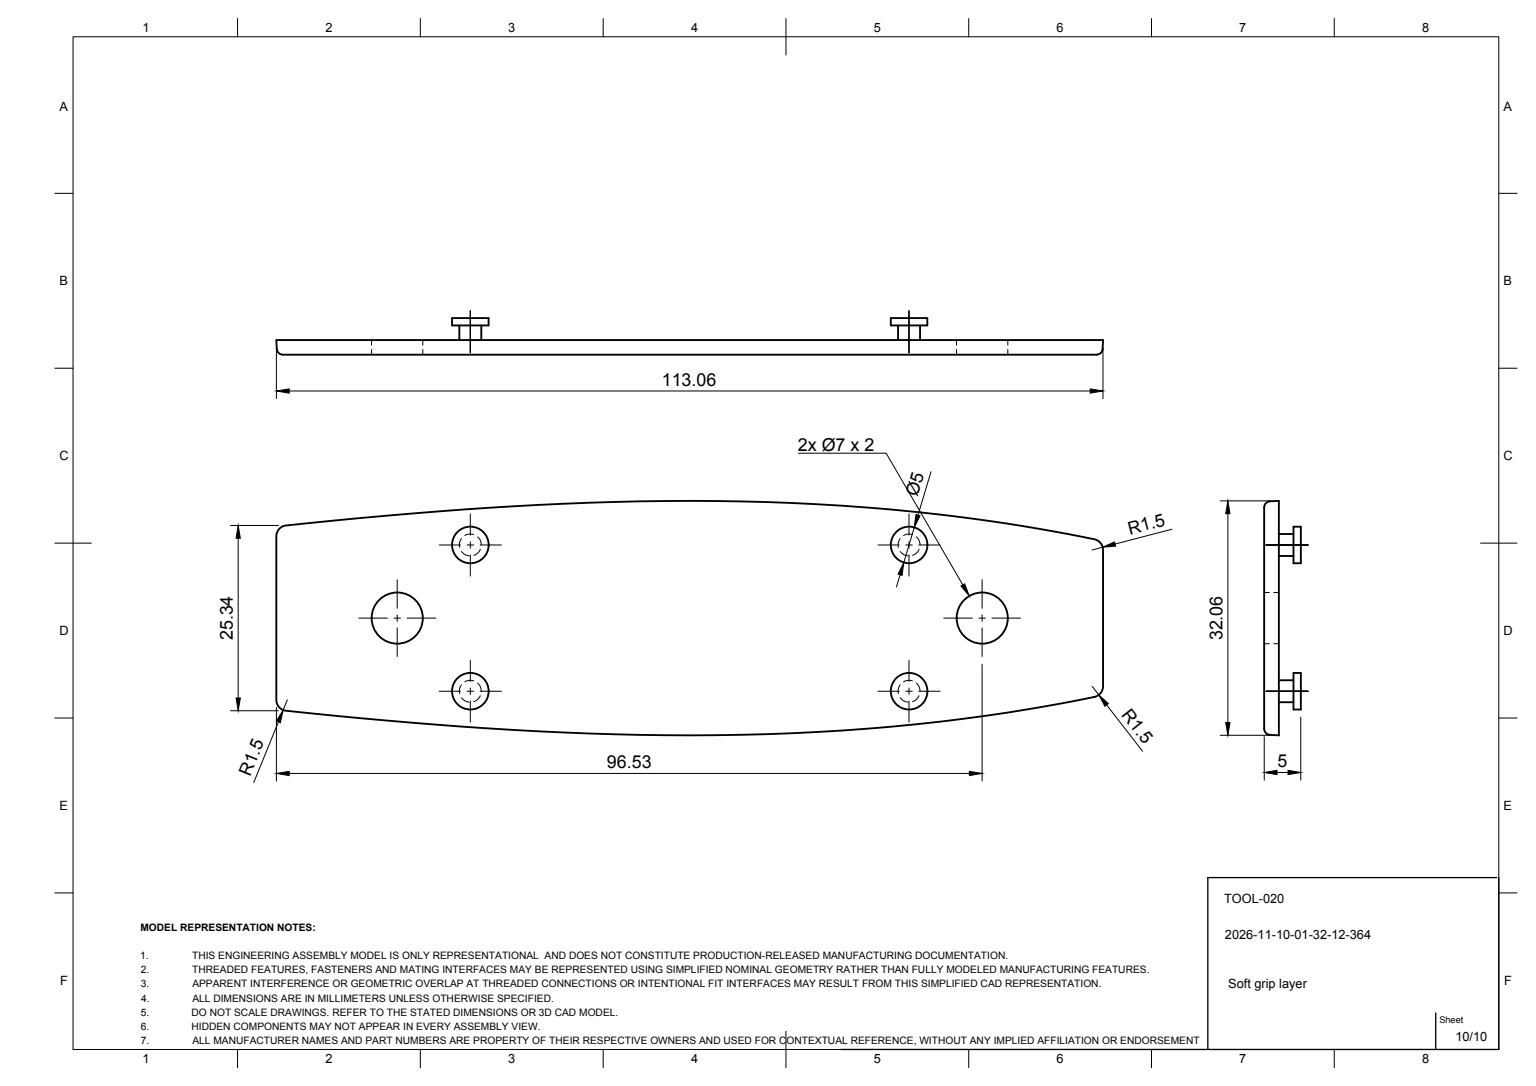
ISO-10303-21;
HEADER;
/* Generated by software containing ST-Developer
 * from STEP Tools, Inc. (www.steptools.com) 
 */

FILE_DESCRIPTION(
/* description */ (''),
/* implementation_level */ '2;1');

FILE_NAME(
/* name */ 'Soft grip layer.step',
/* time_stamp */ '2026-11-10T09:09:39-08:00',
/* author */ (''),
/* organization */ (''),
/* preprocessor_version */ 'ST-DEVELOPER v20.2',
/* originating_system */ 'Autodesk Translation Framework v15.17.0.0',
/* authorisation */ '');

FILE_SCHEMA (('AUTOMOTIVE_DESIGN { 1 0 10303 214 3 1 1 }'));
ENDSEC;

DATA;
#10=MECHANICAL_DESIGN_GEOMETRIC_PRESENTATION_REPRESENTATION('',(#560),#18353);
#155=B_SPLINE_SURFACE_WITH_KNOTS('',3,3,((#12695,#12696,#12697,#12698,#12699),
(#12700,#12701,#12702,#12703,#12704),(#12705,#12706,#12707,#12708,#12709),
(#12710,#12711,#12712,#12713,#12714),(#12715,#12716,#12717,#12718,#12719)),
 .UNSPECIFIED.,.F.,.F.,.F.,(4,1,4),(4,1,4),(0.,0.571428571428571,1.),(0.,
0.0439228984074713,0.102486762950766),.UNSPECIFIED.);
#156=B_SPLINE_SURFACE_WITH_KNOTS('',3,3,((#12742,#12743,#12744,#12745,#12746),
(#12747,#12748,#12749,#12750,#12751),(#12752,#12753,#12754,#12755,#12756),
(#12757,#12758,#12759,#12760,#12761),(#12762,#12763,#12764,#12765,#12766)),
 .UNSPECIFIED.,.F.,.F.,.F.,(4,1,4),(4,1,4),(0.,0.571428571428571,1.),(0.,
0.0439228984484775,0.102486763046448),.UNSPECIFIED.);
#157=B_SPLINE_SURFACE_WITH_KNOTS('',3,3,((#12780,#12781,#12782,#12783,#12784,
#12785),(#12786,#12787,#12788,#12789,#12790,#12791),(#12792,#12793,#12794,
#12795,#12796,#12797),(#12798,#12799,#12800,#12801,#12802,#12803),(#12804,
#12805,#12806,#12807,#12808,#12809)),.UNSPECIFIED.,.F.,.F.,.F.,(4,1,4),
(4,1,1,4),(0.,0.571428571428571,1.),(0.,4.74079765360458,7.9013294226743,
11.061861191744),.UNSPECIFIED.);
#158=B_SPLINE_SURFACE_WITH_KNOTS('',3,3,((#12825,#12826,#12827,#12828,#12829),
(#12830,#12831,#12832,#12833,#12834),(#12835,#12836,#12837,#12838,#12839),
(#12840,#12841,#12842,#12843,#12844),(#12845,#12846,#12847,#12848,#12849)),
 .UNSPECIFIED.,.F.,.F.,.F.,(4,1,4),(4,1,4),(0.,0.571428571428571,1.),(0.,
0.0409389169025732,0.0955241394393374),.UNSPECIFIED.);
#159=B_SPLINE_SURFACE_WITH_KNOTS('',3,3,((#12869,#12870,#12871,#12872,#12873),
(#12874,#12875,#12876,#12877,#12878),(#12879,#12880,#12881,#12882,#12883),
(#12884,#12885,#12886,#12887,#12888),(#12889,#12890,#12891,#12892,#12893)),
 .UNSPECIFIED.,.F.,.F.,.F.,(4,1,4),(4,1,4),(0.,0.571428571428571,1.),(2.31010434703409E-17,
0.054585222365383,0.0955241391394202),.UNSPECIFIED.);
#160=B_SPLINE_SURFACE_WITH_KNOTS('',3,3,((#12907,#12908,#12909,#12910,#12911,
#12912),(#12913,#12914,#12915,#12916,#12917,#12918),(#12919,#12920,#12921,
#12922,#12923,#12924),(#12925,#12926,#12927,#12928,#12929,#12930),(#12931,
#12932,#12933,#12934,#12935,#12936)),.UNSPECIFIED.,.F.,.F.,.F.,(4,1,4),
(4,1,1,4),(0.,0.571428571428571,1.),(1.48308270761676E-15,3.16052629084276,
6.32105258168553,11.0618420179497),.UNSPECIFIED.);
#161=B_SPLINE_SURFACE_WITH_KNOTS('',3,3,((#12961,#12962,#12963,#12964),
(#12965,#12966,#12967,#12968),(#12969,#12970,#12971,#12972),(#12973,#12974,
#12975,#12976),(#12977,#12978,#12979,#12980)),.UNSPECIFIED.,.F.,.F.,.F.,
(4,1,4),(4,4),(0.,0.571428571428571,1.),(-0.0018994230917637,0.12591792480537),
 .UNSPECIFIED.);
#162=B_SPLINE_SURFACE_WITH_KNOTS('',3,3,((#13011,#13012,#13013,#13014),
(#13015,#13016,#13017,#13018),(#13019,#13020,#13021,#13022),(#13023,#13024,
#13025,#13026)),.UNSPECIFIED.,.F.,.F.,.F.,(4,4),(4,4),(0.0105624938889701,
0.988135278219398),(0.,0.624639504152193),.UNSPECIFIED.);
#163=B_SPLINE_SURFACE_WITH_KNOTS('',3,3,((#13036,#13037,#13038,#13039),
(#13040,#13041,#13042,#13043),(#13044,#13045,#13046,#13047),(#13048,#13049,
#13050,#13051),(#13052,#13053,#13054,#13055)),.UNSPECIFIED.,.F.,.F.,.F.,
(4,1,4),(4,4),(0.,0.571428571428571,1.),(-0.00248141748936713,0.125282751535517),
 .UNSPECIFIED.);
#164=B_SPLINE_SURFACE_WITH_KNOTS('',3,3,((#13097,#13098,#13099,#13100),
(#13101,#13102,#13103,#13104),(#13105,#13106,#13107,#13108),(#13109,#13110,
#13111,#13112),(#13113,#13114,#13115,#13116)),.UNSPECIFIED.,.F.,.F.,.F.,
(4,1,4),(4,4),(0.,0.571428571428571,1.),(-0.00183337806924316,0.12591792480537),
 .UNSPECIFIED.);
#165=B_SPLINE_SURFACE_WITH_KNOTS('',3,3,((#13147,#13148,#13149,#13150),
(#13151,#13152,#13153,#13154),(#13155,#13156,#13157,#13158),(#13159,#13160,
#13161,#13162),(#13163,#13164,#13165,#13166)),.UNSPECIFIED.,.F.,.F.,.F.,
(4,1,4),(4,4),(0.,0.571428571428571,1.),(-0.00256306836558615,0.125282751535516),
 .UNSPECIFIED.);
#166=B_SPLINE_SURFACE_WITH_KNOTS('',3,3,((#13205,#13206,#13207,#13208),
(#13209,#13210,#13211,#13212),(#13213,#13214,#13215,#13216),(#13217,#13218,
#13219,#13220)),.UNSPECIFIED.,.F.,.F.,.F.,(4,4),(4,4),(0.0118647217806023,
0.98943750611103),(0.,0.624639504152185),.UNSPECIFIED.);
#355=B_SPLINE_CURVE_WITH_KNOTS('',3,(#12724,#12725,#12726,#12727,#12728),
 .UNSPECIFIED.,.F.,.F.,(4,1,4),(-0.102486762950766,-0.0439228984074713,
0.),.UNSPECIFIED.);
#356=B_SPLINE_CURVE_WITH_KNOTS('',3,(#12731,#12732,#12733,#12734,#12735),
 .UNSPECIFIED.,.F.,.F.,(4,1,4),(0.,0.0439228984074713,0.102486762950766),
 .UNSPECIFIED.);
#357=B_SPLINE_CURVE_WITH_KNOTS('',3,(#12770,#12771,#12772,#12773,#12774),
 .UNSPECIFIED.,.F.,.F.,(4,1,4),(-0.102486763046448,-0.0439228984484775,
0.),.UNSPECIFIED.);
#358=B_SPLINE_CURVE_WITH_KNOTS('',3,(#12775,#12776,#12777,#12778,#12779),
 .UNSPECIFIED.,.F.,.F.,(4,1,4),(0.,0.0439228984484775,0.102486763046448),
 .UNSPECIFIED.);
#359=B_SPLINE_CURVE_WITH_KNOTS('',3,(#12813,#12814,#12815,#12816,#12817,
#12818),.UNSPECIFIED.,.F.,.F.,(4,1,1,4),(-11.061861191744,-7.9013294226743,
-4.74079765360458,0.),.UNSPECIFIED.);
#360=B_SPLINE_CURVE_WITH_KNOTS('',3,(#12819,#12820,#12821,#12822,#12823,
#12824),.UNSPECIFIED.,.F.,.F.,(4,1,1,4),(0.,4.74079765360458,7.9013294226743,
11.061861191744),.UNSPECIFIED.);
#361=B_SPLINE_CURVE_WITH_KNOTS('',3,(#12853,#12854,#12855,#12856,#12857),
 .UNSPECIFIED.,.F.,.F.,(4,1,4),(-0.0955241394393374,-0.0409389169025732,
0.),.UNSPECIFIED.);
#362=B_SPLINE_CURVE_WITH_KNOTS('',3,(#12858,#12859,#12860,#12861,#12862),
 .UNSPECIFIED.,.F.,.F.,(4,1,4),(0.,0.0409389169025732,0.0955241394393374),
 .UNSPECIFIED.);
#363=B_SPLINE_CURVE_WITH_KNOTS('',3,(#12897,#12898,#12899,#12900,#12901),
 .UNSPECIFIED.,.F.,.F.,(4,1,4),(-0.0955241391394202,-0.054585222365383,
-2.31010434703409E-17),.UNSPECIFIED.);
#364=B_SPLINE_CURVE_WITH_KNOTS('',3,(#12902,#12903,#12904,#12905,#12906),
 .UNSPECIFIED.,.F.,.F.,(4,1,4),(2.31010434703409E-17,0.054585222365383,
0.0955241391394202),.UNSPECIFIED.);
#365=B_SPLINE_CURVE_WITH_KNOTS('',3,(#12937,#12938,#12939,#12940,#12941,
#12942),.UNSPECIFIED.,.F.,.F.,(4,1,1,4),(-11.0618420179497,-6.32105258168553,
-3.16052629084276,-1.48308270761676E-15),.UNSPECIFIED.);
#366=B_SPLINE_CURVE_WITH_KNOTS('',3,(#12943,#12944,#12945,#12946,#12947,
#12948),.UNSPECIFIED.,.F.,.F.,(4,1,1,4),(1.48308270761676E-15,3.16052629084276,
6.32105258168553,11.0618420179497),.UNSPECIFIED.);
#367=B_SPLINE_CURVE_WITH_KNOTS('',3,(#12951,#12952,#12953,#12954),
 .UNSPECIFIED.,.F.,.F.,(4,4),(0.00139191041679171,0.12591792480537),
 .UNSPECIFIED.);
#368=B_SPLINE_CURVE_WITH_KNOTS('',3,(#12957,#12958,#12959,#12960),
 .UNSPECIFIED.,.F.,.F.,(4,4),(-0.12591792480537,-0.00139191041679165),
 .UNSPECIFIED.);
#369=B_SPLINE_CURVE_WITH_KNOTS('',3,(#12982,#12983,#12984,#12985),
 .UNSPECIFIED.,.F.,.F.,(4,4),(-0.125267757839186,2.34187669256869E-17),
 .UNSPECIFIED.);
#370=B_SPLINE_CURVE_WITH_KNOTS('',3,(#12986,#12987,#12988,#12989,#12990,
#12991,#12992,#12993,#12994,#12995,#12996,#12997,#12998,#12999,#13000,#13001,
#13002,#13003,#13004,#13005,#13006,#13007,#13008,#13009,#13010),
 .UNSPECIFIED.,.F.,.F.,(4,3,3,3,3,3,3,3,4),(0.,0.0322618866145428,0.0585630993998112,
0.0880157356071287,0.11701919887454,0.14936655709923,0.161132799378038,
0.193259076308563,0.205272292311979),.UNSPECIFIED.);
#371=B_SPLINE_CURVE_WITH_KNOTS('',3,(#13028,#13029,#13030,#13031),
 .UNSPECIFIED.,.F.,.F.,(4,4),(-1.85615411929518E-16,0.12492953807382),
 .UNSPECIFIED.);
#372=B_SPLINE_CURVE_WITH_KNOTS('',3,(#13032,#13033,#13034,#13035),
 .UNSPECIFIED.,.F.,.F.,(4,4),(0.0105624938889701,0.988135278219398),
 .UNSPECIFIED.);
#373=B_SPLINE_CURVE_WITH_KNOTS('',3,(#13057,#13058,#13059,#13060),
 .UNSPECIFIED.,.F.,.F.,(4,4),(-0.125282751535517,-0.000756099764976127),
 .UNSPECIFIED.);
#374=B_SPLINE_CURVE_WITH_KNOTS('',3,(#13061,#13062,#13063,#13064,#13065,
#13066,#13067,#13068,#13069,#13070,#13071,#13072,#13073,#13074,#13075,#13076,
#13077,#13078,#13079,#13080,#13081,#13082,#13083,#13084,#13085,#13086,#13087,
#13088),.UNSPECIFIED.,.F.,.F.,(4,3,3,3,3,3,3,3,3,4),(0.,0.0322721186185131,
0.0586507621648183,0.090893271235385,0.0944607523249211,0.117149429440675,
0.149538018358679,0.168700492523839,0.200858914363656,0.220277485057336),
 .UNSPECIFIED.);
#375=B_SPLINE_CURVE_WITH_KNOTS('',3,(#13092,#13093,#13094,#13095),
 .UNSPECIFIED.,.F.,.F.,(4,4),(0.000756099764976051,0.125282751535516),
 .UNSPECIFIED.);
#376=B_SPLINE_CURVE_WITH_KNOTS('',3,(#13118,#13119,#13120,#13121,#13122,
#13123,#13124,#13125,#13126,#13127,#13128,#13129,#13130,#13131,#13132,#13133,
#13134,#13135,#13136,#13137,#13138,#13139,#13140,#13141,#13142),
 .UNSPECIFIED.,.F.,.F.,(4,3,3,3,3,3,3,3,4),(-1.38777878078145E-17,0.0322740250441291,
0.0586501551213245,0.0880475535304867,0.117148640042868,0.149495851515852,
0.161204029299056,0.193312734374797,0.205276387553207),.UNSPECIFIED.);
#377=B_SPLINE_CURVE_WITH_KNOTS('',3,(#13143,#13144,#13145,#13146),
 .UNSPECIFIED.,.F.,.F.,(4,4),(5.20417042793042E-18,0.125267757839184),
 .UNSPECIFIED.);
#378=B_SPLINE_CURVE_WITH_KNOTS('',3,(#13168,#13169,#13170,#13171),
 .UNSPECIFIED.,.F.,.F.,(4,4),(-0.124929538073804,-1.0547118733939E-15),
 .UNSPECIFIED.);
#379=B_SPLINE_CURVE_WITH_KNOTS('',3,(#13172,#13173,#13174,#13175,#13176,
#13177,#13178,#13179,#13180,#13181,#13182,#13183,#13184,#13185,#13186,#13187,
#13188,#13189,#13190,#13191,#13192,#13193,#13194,#13195,#13196,#13197,#13198,
#13199),.UNSPECIFIED.,.F.,.F.,(4,3,3,3,3,3,3,3,3,4),(0.,0.0322648940196546,
0.0586047006713273,0.0908498906869236,0.0944423330072586,0.117077542275299,
0.149464200283694,0.168660330271145,0.200827593216919,0.220275105166519),
 .UNSPECIFIED.);
#380=B_SPLINE_CURVE_WITH_KNOTS('',3,(#13201,#13202,#13203,#13204),
 .UNSPECIFIED.,.F.,.F.,(4,4),(0.0118647217806024,0.98943750611103),
 .UNSPECIFIED.);
#542=SHAPE_REPRESENTATION_RELATIONSHIP('SRR','None',#18403,#551);
#551=ADVANCED_BREP_SHAPE_REPRESENTATION('',(#569),#18349);
#560=STYLED_ITEM('',(#18460),#569);
#569=MANIFOLD_SOLID_BREP('Body1',#6491);
#620=FACE_BOUND('',#1438,.T.);
#621=FACE_BOUND('',#1442,.T.);
#622=FACE_BOUND('',#1446,.T.);
#623=FACE_BOUND('',#1450,.T.);
#624=FACE_BOUND('',#1470,.T.);
#625=FACE_BOUND('',#1471,.T.);
#626=FACE_BOUND('',#1476,.T.);
#627=FACE_BOUND('',#1477,.T.);
#628=FACE_BOUND('',#1478,.T.);
#629=FACE_BOUND('',#1479,.T.);
#630=FACE_BOUND('',#1480,.T.);
#631=FACE_BOUND('',#1481,.T.);
#750=PLANE('',#6903);
#751=PLANE('',#6908);
#752=PLANE('',#6909);
#753=PLANE('',#6914);
#754=PLANE('',#6915);
#755=PLANE('',#6920);
#756=PLANE('',#6921);
#757=PLANE('',#6926);
#758=PLANE('',#6945);
#759=PLANE('',#6946);
#760=PLANE('',#6947);
#761=PLANE('',#6948);
#1017=FACE_OUTER_BOUND('',#1435,.T.);
#1018=FACE_OUTER_BOUND('',#1436,.T.);
#1019=FACE_OUTER_BOUND('',#1437,.T.);
#1020=FACE_OUTER_BOUND('',#1439,.T.);
#1021=FACE_OUTER_BOUND('',#1440,.T.);
#1022=FACE_OUTER_BOUND('',#1441,.T.);
#1023=FACE_OUTER_BOUND('',#1443,.T.);
#1024=FACE_OUTER_BOUND('',#1444,.T.);
#1025=FACE_OUTER_BOUND('',#1445,.T.);
#1026=FACE_OUTER_BOUND('',#1447,.T.);
#1027=FACE_OUTER_BOUND('',#1448,.T.);
#1028=FACE_OUTER_BOUND('',#1449,.T.);
#1029=FACE_OUTER_BOUND('',#1451,.T.);
#1030=FACE_OUTER_BOUND('',#1452,.T.);
#1031=FACE_OUTER_BOUND('',#1453,.T.);
#1032=FACE_OUTER_BOUND('',#1454,.T.);
#1033=FACE_OUTER_BOUND('',#1455,.T.);
#1034=FACE_OUTER_BOUND('',#1456,.T.);
#1035=FACE_OUTER_BOUND('',#1457,.T.);
#1036=FACE_OUTER_BOUND('',#1458,.T.);
#1037=FACE_OUTER_BOUND('',#1459,.T.);
#1038=FACE_OUTER_BOUND('',#1460,.T.);
#1039=FACE_OUTER_BOUND('',#1461,.T.);
#1040=FACE_OUTER_BOUND('',#1462,.T.);
#1041=FACE_OUTER_BOUND('',#1463,.T.);
#1042=FACE_OUTER_BOUND('',#1464,.T.);
#1043=FACE_OUTER_BOUND('',#1465,.T.);
#1044=FACE_OUTER_BOUND('',#1466,.T.);
#1045=FACE_OUTER_BOUND('',#1467,.T.);
#1046=FACE_OUTER_BOUND('',#1468,.T.);
#1047=FACE_OUTER_BOUND('',#1469,.T.);
#1048=FACE_OUTER_BOUND('',#1472,.T.);
#1049=FACE_OUTER_BOUND('',#1473,.T.);
#1050=FACE_OUTER_BOUND('',#1474,.T.);
#1051=FACE_OUTER_BOUND('',#1475,.T.);
#1052=FACE_OUTER_BOUND('',#1482,.T.);
#1435=EDGE_LOOP('',(#5278,#5279,#5280,#5281));
#1436=EDGE_LOOP('',(#5282,#5283,#5284,#5285));
#1437=EDGE_LOOP('',(#5286));
#1438=EDGE_LOOP('',(#5287));
#1439=EDGE_LOOP('',(#5288,#5289,#5290,#5291));
#1440=EDGE_LOOP('',(#5292));
#1441=EDGE_LOOP('',(#5293));
#1442=EDGE_LOOP('',(#5294));
#1443=EDGE_LOOP('',(#5295,#5296,#5297,#5298));
#1444=EDGE_LOOP('',(#5299));
#1445=EDGE_LOOP('',(#5300));
#1446=EDGE_LOOP('',(#5301));
#1447=EDGE_LOOP('',(#5302,#5303,#5304,#5305));
#1448=EDGE_LOOP('',(#5306));
#1449=EDGE_LOOP('',(#5307));
#1450=EDGE_LOOP('',(#5308));
#1451=EDGE_LOOP('',(#5309,#5310,#5311,#5312));
#1452=EDGE_LOOP('',(#5313));
#1453=EDGE_LOOP('',(#5314,#5315,#5316,#5317));
#1454=EDGE_LOOP('',(#5318,#5319,#5320,#5321));
#1455=EDGE_LOOP('',(#5322,#5323,#5324,#5325));
#1456=EDGE_LOOP('',(#5326,#5327,#5328,#5329));
#1457=EDGE_LOOP('',(#5330,#5331,#5332,#5333));
#1458=EDGE_LOOP('',(#5334,#5335,#5336,#5337));
#1459=EDGE_LOOP('',(#5338,#5339,#5340,#5341));
#1460=EDGE_LOOP('',(#5342,#5343,#5344,#5345));
#1461=EDGE_LOOP('',(#5346,#5347,#5348,#5349));
#1462=EDGE_LOOP('',(#5350,#5351,#5352,#5353));
#1463=EDGE_LOOP('',(#5354,#5355,#5356,#5357));
#1464=EDGE_LOOP('',(#5358,#5359,#5360,#5361));
#1465=EDGE_LOOP('',(#5362,#5363,#5364,#5365));
#1466=EDGE_LOOP('',(#5366,#5367,#5368,#5369));
#1467=EDGE_LOOP('',(#5370,#5371,#5372,#5373));
#1468=EDGE_LOOP('',(#5374,#5375,#5376,#5377));
#1469=EDGE_LOOP('',(#5378,#5379,#5380,#5381,#5382,#5383,#5384,#5385));
#1470=EDGE_LOOP('',(#5386));
#1471=EDGE_LOOP('',(#5387));
#1472=EDGE_LOOP('',(#5388,#5389,#5390,#5391));
#1473=EDGE_LOOP('',(#5392,#5393,#5394,#5395));
#1474=EDGE_LOOP('',(#5396,#5397,#5398,#5399));
#1475=EDGE_LOOP('',(#5400,#5401,#5402,#5403,#5404,#5405,#5406,#5407));
#1476=EDGE_LOOP('',(#5408));
#1477=EDGE_LOOP('',(#5409));
#1478=EDGE_LOOP('',(#5410));
#1479=EDGE_LOOP('',(#5411));
#1480=EDGE_LOOP('',(#5412));
#1481=EDGE_LOOP('',(#5413));
#1482=EDGE_LOOP('',(#5414,#5415,#5416,#5417));
#1869=LINE('',#12631,#2273);
#1870=LINE('',#12637,#2274);
#1871=LINE('',#12647,#2275);
#1872=LINE('',#12657,#2276);
#1873=LINE('',#12667,#2277);
#1874=LINE('',#12677,#2278);
#1875=LINE('',#12681,#2279);
#1876=LINE('',#12685,#2280);
#1877=LINE('',#12689,#2281);
#1878=LINE('',#12693,#2282);
#1879=LINE('',#12740,#2283);
#1880=LINE('',#12741,#2284);
#1881=LINE('',#12867,#2285);
#1882=LINE('',#12868,#2286);
#1883=LINE('',#12956,#2287);
#1884=LINE('',#13096,#2288);
#2273=VECTOR('',#7968,0.35);
#2274=VECTOR('',#7975,0.35);
#2275=VECTOR('',#7988,0.25);
#2276=VECTOR('',#8001,0.25);
#2277=VECTOR('',#8014,0.25);
#2278=VECTOR('',#8027,0.25);
#2279=VECTOR('',#8032,0.15);
#2280=VECTOR('',#8037,0.15);
#2281=VECTOR('',#8042,0.15);
#2282=VECTOR('',#8047,0.15);
#2283=VECTOR('',#8058,1.);
#2284=VECTOR('',#8059,1.);
#2285=VECTOR('',#8070,1.);
#2286=VECTOR('',#8071,1.);
#2287=VECTOR('',#8076,1.);
#2288=VECTOR('',#8081,1.);
#2522=CIRCLE('',#6898,0.35);
#2523=CIRCLE('',#6899,0.35);
#2524=CIRCLE('',#6901,0.35);
#2525=CIRCLE('',#6902,0.35);
#2526=CIRCLE('',#6904,0.25);
#2527=CIRCLE('',#6905,0.15);
#2528=CIRCLE('',#6907,0.25);
#2529=CIRCLE('',#6910,0.25);
#2530=CIRCLE('',#6911,0.15);
#2531=CIRCLE('',#6913,0.25);
#2532=CIRCLE('',#6916,0.25);
#2533=CIRCLE('',#6917,0.15);
#2534=CIRCLE('',#6919,0.25);
#2535=CIRCLE('',#6922,0.25);
#2536=CIRCLE('',#6923,0.15);
#2537=CIRCLE('',#6925,0.25);
#2538=CIRCLE('',#6928,0.15);
#2539=CIRCLE('',#6930,0.15);
#2540=CIRCLE('',#6932,0.15);
#2541=CIRCLE('',#6934,0.15);
#2542=CIRCLE('',#6935,0.0800000000000001);
#2543=CIRCLE('',#6936,0.0799999999999999);
#2544=CIRCLE('',#6938,0.0800000000000001);
#2545=CIRCLE('',#6939,0.0799999999999998);
#2546=CIRCLE('',#6940,0.0800000000000001);
#2547=CIRCLE('',#6941,0.0800000000000001);
#2548=CIRCLE('',#6943,0.0800000000000001);
#2549=CIRCLE('',#6944,0.0799999999999998);
#2939=VERTEX_POINT('',#12628);
#2940=VERTEX_POINT('',#12630);
#2941=VERTEX_POINT('',#12634);
#2942=VERTEX_POINT('',#12636);
#2943=VERTEX_POINT('',#12640);
#2944=VERTEX_POINT('',#12642);
#2945=VERTEX_POINT('',#12645);
#2946=VERTEX_POINT('',#12650);
#2947=VERTEX_POINT('',#12652);
#2948=VERTEX_POINT('',#12655);
#2949=VERTEX_POINT('',#12660);
#2950=VERTEX_POINT('',#12662);
#2951=VERTEX_POINT('',#12665);
#2952=VERTEX_POINT('',#12670);
#2953=VERTEX_POINT('',#12672);
#2954=VERTEX_POINT('',#12675);
#2955=VERTEX_POINT('',#12680);
#2956=VERTEX_POINT('',#12684);
#2957=VERTEX_POINT('',#12688);
#2958=VERTEX_POINT('',#12692);
#2959=VERTEX_POINT('',#12720);
#2960=VERTEX_POINT('',#12721);
#2961=VERTEX_POINT('',#12723);
#2962=VERTEX_POINT('',#12729);
#2963=VERTEX_POINT('',#12737);
#2964=VERTEX_POINT('',#12738);
#2965=VERTEX_POINT('',#12767);
#2966=VERTEX_POINT('',#12768);
#2967=VERTEX_POINT('',#12810);
#2968=VERTEX_POINT('',#12811);
#2969=VERTEX_POINT('',#12850);
#2970=VERTEX_POINT('',#12851);
#2971=VERTEX_POINT('',#12864);
#2972=VERTEX_POINT('',#12865);
#2973=VERTEX_POINT('',#12894);
#2974=VERTEX_POINT('',#12895);
#2975=VERTEX_POINT('',#12950);
#2976=VERTEX_POINT('',#12955);
#2977=VERTEX_POINT('',#12981);
#2978=VERTEX_POINT('',#13027);
#2979=VERTEX_POINT('',#13056);
#2980=VERTEX_POINT('',#13091);
#2981=VERTEX_POINT('',#13117);
#2982=VERTEX_POINT('',#13167);
#3756=EDGE_CURVE('',#2939,#2939,#2522,.T.);
#3757=EDGE_CURVE('',#2939,#2940,#1869,.T.);
#3758=EDGE_CURVE('',#2940,#2940,#2523,.T.);
#3759=EDGE_CURVE('',#2941,#2941,#2524,.T.);
#3760=EDGE_CURVE('',#2941,#2942,#1870,.T.);
#3761=EDGE_CURVE('',#2942,#2942,#2525,.T.);
#3762=EDGE_CURVE('',#2943,#2943,#2526,.T.);
#3763=EDGE_CURVE('',#2944,#2944,#2527,.T.);
#3764=EDGE_CURVE('',#2945,#2945,#2528,.T.);
#3765=EDGE_CURVE('',#2945,#2943,#1871,.T.);
#3766=EDGE_CURVE('',#2946,#2946,#2529,.T.);
#3767=EDGE_CURVE('',#2947,#2947,#2530,.T.);
#3768=EDGE_CURVE('',#2948,#2948,#2531,.T.);
#3769=EDGE_CURVE('',#2948,#2946,#1872,.T.);
#3770=EDGE_CURVE('',#2949,#2949,#2532,.T.);
#3771=EDGE_CURVE('',#2950,#2950,#2533,.T.);
#3772=EDGE_CURVE('',#2951,#2951,#2534,.T.);
#3773=EDGE_CURVE('',#2951,#2949,#1873,.T.);
#3774=EDGE_CURVE('',#2952,#2952,#2535,.T.);
#3775=EDGE_CURVE('',#2953,#2953,#2536,.T.);
#3776=EDGE_CURVE('',#2954,#2954,#2537,.T.);
#3777=EDGE_CURVE('',#2954,#2952,#1874,.T.);
#3778=EDGE_CURVE('',#2944,#2955,#1875,.T.);
#3779=EDGE_CURVE('',#2955,#2955,#2538,.T.);
#3780=EDGE_CURVE('',#2947,#2956,#1876,.T.);
#3781=EDGE_CURVE('',#2956,#2956,#2539,.T.);
#3782=EDGE_CURVE('',#2950,#2957,#1877,.T.);
#3783=EDGE_CURVE('',#2957,#2957,#2540,.T.);
#3784=EDGE_CURVE('',#2953,#2958,#1878,.T.);
#3785=EDGE_CURVE('',#2958,#2958,#2541,.T.);
#3786=EDGE_CURVE('',#2959,#2960,#2542,.T.);
#3787=EDGE_CURVE('',#2960,#2961,#355,.T.);
#3788=EDGE_CURVE('',#2961,#2962,#2543,.T.);
#3789=EDGE_CURVE('',#2962,#2959,#356,.T.);
#3790=EDGE_CURVE('',#2963,#2964,#2544,.T.);
#3791=EDGE_CURVE('',#2964,#2960,#1879,.T.);
#3792=EDGE_CURVE('',#2959,#2963,#1880,.T.);
#3793=EDGE_CURVE('',#2965,#2966,#2545,.T.);
#3794=EDGE_CURVE('',#2966,#2964,#357,.T.);
#3795=EDGE_CURVE('',#2963,#2965,#358,.T.);
#3796=EDGE_CURVE('',#2967,#2968,#2546,.T.);
#3797=EDGE_CURVE('',#2968,#2966,#359,.T.);
#3798=EDGE_CURVE('',#2965,#2967,#360,.T.);
#3799=EDGE_CURVE('',#2969,#2970,#2547,.T.);
#3800=EDGE_CURVE('',#2970,#2968,#361,.T.);
#3801=EDGE_CURVE('',#2967,#2969,#362,.T.);
#3802=EDGE_CURVE('',#2971,#2972,#2548,.T.);
#3803=EDGE_CURVE('',#2972,#2970,#1881,.T.);
#3804=EDGE_CURVE('',#2969,#2971,#1882,.T.);
#3805=EDGE_CURVE('',#2973,#2974,#2549,.T.);
#3806=EDGE_CURVE('',#2974,#2972,#363,.T.);
#3807=EDGE_CURVE('',#2971,#2973,#364,.T.);
#3808=EDGE_CURVE('',#2961,#2974,#365,.T.);
#3809=EDGE_CURVE('',#2973,#2962,#366,.T.);
#3810=EDGE_CURVE('',#2975,#2972,#367,.T.);
#3811=EDGE_CURVE('',#2976,#2975,#1883,.T.);
#3812=EDGE_CURVE('',#2970,#2976,#368,.T.);
#3813=EDGE_CURVE('',#2974,#2977,#369,.T.);
#3814=EDGE_CURVE('',#2977,#2975,#370,.T.);
#3815=EDGE_CURVE('',#2978,#2961,#371,.T.);
#3816=EDGE_CURVE('',#2977,#2978,#372,.T.);
#3817=EDGE_CURVE('',#2960,#2979,#373,.T.);
#3818=EDGE_CURVE('',#2979,#2978,#374,.T.);
#3819=EDGE_CURVE('',#2980,#2964,#375,.T.);
#3820=EDGE_CURVE('',#2979,#2980,#1884,.T.);
#3821=EDGE_CURVE('',#2976,#2981,#376,.T.);
#3822=EDGE_CURVE('',#2981,#2968,#377,.T.);
#3823=EDGE_CURVE('',#2966,#2982,#378,.T.);
#3824=EDGE_CURVE('',#2982,#2980,#379,.T.);
#3825=EDGE_CURVE('',#2982,#2981,#380,.T.);
#5278=ORIENTED_EDGE('',*,*,#3756,.F.);
#5279=ORIENTED_EDGE('',*,*,#3757,.T.);
#5280=ORIENTED_EDGE('',*,*,#3758,.F.);
#5281=ORIENTED_EDGE('',*,*,#3757,.F.);
#5282=ORIENTED_EDGE('',*,*,#3759,.F.);
#5283=ORIENTED_EDGE('',*,*,#3760,.T.);
#5284=ORIENTED_EDGE('',*,*,#3761,.F.);
#5285=ORIENTED_EDGE('',*,*,#3760,.F.);
#5286=ORIENTED_EDGE('',*,*,#3762,.T.);
#5287=ORIENTED_EDGE('',*,*,#3763,.T.);
#5288=ORIENTED_EDGE('',*,*,#3764,.F.);
#5289=ORIENTED_EDGE('',*,*,#3765,.T.);
#5290=ORIENTED_EDGE('',*,*,#3762,.F.);
#5291=ORIENTED_EDGE('',*,*,#3765,.F.);
#5292=ORIENTED_EDGE('',*,*,#3764,.T.);
#5293=ORIENTED_EDGE('',*,*,#3766,.T.);
#5294=ORIENTED_EDGE('',*,*,#3767,.T.);
#5295=ORIENTED_EDGE('',*,*,#3768,.F.);
#5296=ORIENTED_EDGE('',*,*,#3769,.T.);
#5297=ORIENTED_EDGE('',*,*,#3766,.F.);
#5298=ORIENTED_EDGE('',*,*,#3769,.F.);
#5299=ORIENTED_EDGE('',*,*,#3768,.T.);
#5300=ORIENTED_EDGE('',*,*,#3770,.T.);
#5301=ORIENTED_EDGE('',*,*,#3771,.T.);
#5302=ORIENTED_EDGE('',*,*,#3772,.F.);
#5303=ORIENTED_EDGE('',*,*,#3773,.T.);
#5304=ORIENTED_EDGE('',*,*,#3770,.F.);
#5305=ORIENTED_EDGE('',*,*,#3773,.F.);
#5306=ORIENTED_EDGE('',*,*,#3772,.T.);
#5307=ORIENTED_EDGE('',*,*,#3774,.T.);
#5308=ORIENTED_EDGE('',*,*,#3775,.T.);
#5309=ORIENTED_EDGE('',*,*,#3776,.F.);
#5310=ORIENTED_EDGE('',*,*,#3777,.T.);
#5311=ORIENTED_EDGE('',*,*,#3774,.F.);
#5312=ORIENTED_EDGE('',*,*,#3777,.F.);
#5313=ORIENTED_EDGE('',*,*,#3776,.T.);
#5314=ORIENTED_EDGE('',*,*,#3763,.F.);
#5315=ORIENTED_EDGE('',*,*,#3778,.T.);
#5316=ORIENTED_EDGE('',*,*,#3779,.F.);
#5317=ORIENTED_EDGE('',*,*,#3778,.F.);
#5318=ORIENTED_EDGE('',*,*,#3767,.F.);
#5319=ORIENTED_EDGE('',*,*,#3780,.T.);
#5320=ORIENTED_EDGE('',*,*,#3781,.F.);
#5321=ORIENTED_EDGE('',*,*,#3780,.F.);
#5322=ORIENTED_EDGE('',*,*,#3771,.F.);
#5323=ORIENTED_EDGE('',*,*,#3782,.T.);
#5324=ORIENTED_EDGE('',*,*,#3783,.F.);
#5325=ORIENTED_EDGE('',*,*,#3782,.F.);
#5326=ORIENTED_EDGE('',*,*,#3775,.F.);
#5327=ORIENTED_EDGE('',*,*,#3784,.T.);
#5328=ORIENTED_EDGE('',*,*,#3785,.F.);
#5329=ORIENTED_EDGE('',*,*,#3784,.F.);
#5330=ORIENTED_EDGE('',*,*,#3786,.T.);
#5331=ORIENTED_EDGE('',*,*,#3787,.T.);
#5332=ORIENTED_EDGE('',*,*,#3788,.T.);
#5333=ORIENTED_EDGE('',*,*,#3789,.T.);
#5334=ORIENTED_EDGE('',*,*,#3790,.T.);
#5335=ORIENTED_EDGE('',*,*,#3791,.T.);
#5336=ORIENTED_EDGE('',*,*,#3786,.F.);
#5337=ORIENTED_EDGE('',*,*,#3792,.T.);
#5338=ORIENTED_EDGE('',*,*,#3793,.T.);
#5339=ORIENTED_EDGE('',*,*,#3794,.T.);
#5340=ORIENTED_EDGE('',*,*,#3790,.F.);
#5341=ORIENTED_EDGE('',*,*,#3795,.T.);
#5342=ORIENTED_EDGE('',*,*,#3796,.T.);
#5343=ORIENTED_EDGE('',*,*,#3797,.T.);
#5344=ORIENTED_EDGE('',*,*,#3793,.F.);
#5345=ORIENTED_EDGE('',*,*,#3798,.T.);
#5346=ORIENTED_EDGE('',*,*,#3799,.T.);
#5347=ORIENTED_EDGE('',*,*,#3800,.T.);
#5348=ORIENTED_EDGE('',*,*,#3796,.F.);
#5349=ORIENTED_EDGE('',*,*,#3801,.T.);
#5350=ORIENTED_EDGE('',*,*,#3802,.T.);
#5351=ORIENTED_EDGE('',*,*,#3803,.T.);
#5352=ORIENTED_EDGE('',*,*,#3799,.F.);
#5353=ORIENTED_EDGE('',*,*,#3804,.T.);
#5354=ORIENTED_EDGE('',*,*,#3805,.T.);
#5355=ORIENTED_EDGE('',*,*,#3806,.T.);
#5356=ORIENTED_EDGE('',*,*,#3802,.F.);
#5357=ORIENTED_EDGE('',*,*,#3807,.T.);
#5358=ORIENTED_EDGE('',*,*,#3788,.F.);
#5359=ORIENTED_EDGE('',*,*,#3808,.T.);
#5360=ORIENTED_EDGE('',*,*,#3805,.F.);
#5361=ORIENTED_EDGE('',*,*,#3809,.T.);
#5362=ORIENTED_EDGE('',*,*,#3803,.F.);
#5363=ORIENTED_EDGE('',*,*,#3810,.F.);
#5364=ORIENTED_EDGE('',*,*,#3811,.F.);
#5365=ORIENTED_EDGE('',*,*,#3812,.F.);
#5366=ORIENTED_EDGE('',*,*,#3806,.F.);
#5367=ORIENTED_EDGE('',*,*,#3813,.T.);
#5368=ORIENTED_EDGE('',*,*,#3814,.T.);
#5369=ORIENTED_EDGE('',*,*,#3810,.T.);
#5370=ORIENTED_EDGE('',*,*,#3808,.F.);
#5371=ORIENTED_EDGE('',*,*,#3815,.F.);
#5372=ORIENTED_EDGE('',*,*,#3816,.F.);
#5373=ORIENTED_EDGE('',*,*,#3813,.F.);
#5374=ORIENTED_EDGE('',*,*,#3787,.F.);
#5375=ORIENTED_EDGE('',*,*,#3817,.T.);
#5376=ORIENTED_EDGE('',*,*,#3818,.T.);
#5377=ORIENTED_EDGE('',*,*,#3815,.T.);
#5378=ORIENTED_EDGE('',*,*,#3789,.F.);
#5379=ORIENTED_EDGE('',*,*,#3809,.F.);
#5380=ORIENTED_EDGE('',*,*,#3807,.F.);
#5381=ORIENTED_EDGE('',*,*,#3804,.F.);
#5382=ORIENTED_EDGE('',*,*,#3801,.F.);
#5383=ORIENTED_EDGE('',*,*,#3798,.F.);
#5384=ORIENTED_EDGE('',*,*,#3795,.F.);
#5385=ORIENTED_EDGE('',*,*,#3792,.F.);
#5386=ORIENTED_EDGE('',*,*,#3756,.T.);
#5387=ORIENTED_EDGE('',*,*,#3759,.T.);
#5388=ORIENTED_EDGE('',*,*,#3791,.F.);
#5389=ORIENTED_EDGE('',*,*,#3819,.F.);
#5390=ORIENTED_EDGE('',*,*,#3820,.F.);
#5391=ORIENTED_EDGE('',*,*,#3817,.F.);
#5392=ORIENTED_EDGE('',*,*,#3800,.F.);
#5393=ORIENTED_EDGE('',*,*,#3812,.T.);
#5394=ORIENTED_EDGE('',*,*,#3821,.T.);
#5395=ORIENTED_EDGE('',*,*,#3822,.T.);
#5396=ORIENTED_EDGE('',*,*,#3794,.F.);
#5397=ORIENTED_EDGE('',*,*,#3823,.T.);
#5398=ORIENTED_EDGE('',*,*,#3824,.T.);
#5399=ORIENTED_EDGE('',*,*,#3819,.T.);
#5400=ORIENTED_EDGE('',*,*,#3818,.F.);
#5401=ORIENTED_EDGE('',*,*,#3820,.T.);
#5402=ORIENTED_EDGE('',*,*,#3824,.F.);
#5403=ORIENTED_EDGE('',*,*,#3825,.T.);
#5404=ORIENTED_EDGE('',*,*,#3821,.F.);
#5405=ORIENTED_EDGE('',*,*,#3811,.T.);
#5406=ORIENTED_EDGE('',*,*,#3814,.F.);
#5407=ORIENTED_EDGE('',*,*,#3816,.T.);
#5408=ORIENTED_EDGE('',*,*,#3758,.T.);
#5409=ORIENTED_EDGE('',*,*,#3761,.T.);
#5410=ORIENTED_EDGE('',*,*,#3779,.T.);
#5411=ORIENTED_EDGE('',*,*,#3781,.T.);
#5412=ORIENTED_EDGE('',*,*,#3783,.T.);
#5413=ORIENTED_EDGE('',*,*,#3785,.T.);
#5414=ORIENTED_EDGE('',*,*,#3797,.F.);
#5415=ORIENTED_EDGE('',*,*,#3822,.F.);
#5416=ORIENTED_EDGE('',*,*,#3825,.F.);
#5417=ORIENTED_EDGE('',*,*,#3823,.F.);
#6024=CYLINDRICAL_SURFACE('',#6897,0.35);
#6025=CYLINDRICAL_SURFACE('',#6900,0.35);
#6026=CYLINDRICAL_SURFACE('',#6906,0.25);
#6027=CYLINDRICAL_SURFACE('',#6912,0.25);
#6028=CYLINDRICAL_SURFACE('',#6918,0.25);
#6029=CYLINDRICAL_SURFACE('',#6924,0.25);
#6030=CYLINDRICAL_SURFACE('',#6927,0.15);
#6031=CYLINDRICAL_SURFACE('',#6929,0.15);
#6032=CYLINDRICAL_SURFACE('',#6931,0.15);
#6033=CYLINDRICAL_SURFACE('',#6933,0.15);
#6034=CYLINDRICAL_SURFACE('',#6937,0.08);
#6035=CYLINDRICAL_SURFACE('',#6942,0.08);
#6348=ADVANCED_FACE('',(#1017),#6024,.F.);
#6349=ADVANCED_FACE('',(#1018),#6025,.F.);
#6350=ADVANCED_FACE('',(#1019,#620),#750,.T.);
#6351=ADVANCED_FACE('',(#1020),#6026,.T.);
#6352=ADVANCED_FACE('',(#1021),#751,.F.);
#6353=ADVANCED_FACE('',(#1022,#621),#752,.T.);
#6354=ADVANCED_FACE('',(#1023),#6027,.T.);
#6355=ADVANCED_FACE('',(#1024),#753,.F.);
#6356=ADVANCED_FACE('',(#1025,#622),#754,.T.);
#6357=ADVANCED_FACE('',(#1026),#6028,.T.);
#6358=ADVANCED_FACE('',(#1027),#755,.F.);
#6359=ADVANCED_FACE('',(#1028,#623),#756,.T.);
#6360=ADVANCED_FACE('',(#1029),#6029,.T.);
#6361=ADVANCED_FACE('',(#1030),#757,.F.);
#6362=ADVANCED_FACE('',(#1031),#6030,.T.);
#6363=ADVANCED_FACE('',(#1032),#6031,.T.);
#6364=ADVANCED_FACE('',(#1033),#6032,.T.);
#6365=ADVANCED_FACE('',(#1034),#6033,.T.);
#6366=ADVANCED_FACE('',(#1035),#155,.F.);
#6367=ADVANCED_FACE('',(#1036),#6034,.T.);
#6368=ADVANCED_FACE('',(#1037),#156,.F.);
#6369=ADVANCED_FACE('',(#1038),#157,.F.);
#6370=ADVANCED_FACE('',(#1039),#158,.F.);
#6371=ADVANCED_FACE('',(#1040),#6035,.T.);
#6372=ADVANCED_FACE('',(#1041),#159,.F.);
#6373=ADVANCED_FACE('',(#1042),#160,.F.);
#6374=ADVANCED_FACE('',(#1043),#758,.F.);
#6375=ADVANCED_FACE('',(#1044),#161,.F.);
#6376=ADVANCED_FACE('',(#1045),#162,.F.);
#6377=ADVANCED_FACE('',(#1046),#163,.F.);
#6378=ADVANCED_FACE('',(#1047,#624,#625),#759,.T.);
#6379=ADVANCED_FACE('',(#1048),#760,.F.);
#6380=ADVANCED_FACE('',(#1049),#164,.F.);
#6381=ADVANCED_FACE('',(#1050),#165,.F.);
#6382=ADVANCED_FACE('',(#1051,#626,#627,#628,#629,#630,#631),#761,.F.);
#6383=ADVANCED_FACE('',(#1052),#166,.F.);
#6491=CLOSED_SHELL('',(#6348,#6349,#6350,#6351,#6352,#6353,#6354,#6355,
#6356,#6357,#6358,#6359,#6360,#6361,#6362,#6363,#6364,#6365,#6366,#6367,
#6368,#6369,#6370,#6371,#6372,#6373,#6374,#6375,#6376,#6377,#6378,#6379,
#6380,#6381,#6382,#6383));
#6896=AXIS2_PLACEMENT_3D('',#12626,#7962,#7963);
#6897=AXIS2_PLACEMENT_3D('',#12627,#7964,#7965);
#6898=AXIS2_PLACEMENT_3D('',#12629,#7966,#7967);
#6899=AXIS2_PLACEMENT_3D('',#12632,#7969,#7970);
#6900=AXIS2_PLACEMENT_3D('',#12633,#7971,#7972);
#6901=AXIS2_PLACEMENT_3D('',#12635,#7973,#7974);
#6902=AXIS2_PLACEMENT_3D('',#12638,#7976,#7977);
#6903=AXIS2_PLACEMENT_3D('',#12639,#7978,#7979);
#6904=AXIS2_PLACEMENT_3D('',#12641,#7980,#7981);
#6905=AXIS2_PLACEMENT_3D('',#12643,#7982,#7983);
#6906=AXIS2_PLACEMENT_3D('',#12644,#7984,#7985);
#6907=AXIS2_PLACEMENT_3D('',#12646,#7986,#7987);
#6908=AXIS2_PLACEMENT_3D('',#12648,#7989,#7990);
#6909=AXIS2_PLACEMENT_3D('',#12649,#7991,#7992);
#6910=AXIS2_PLACEMENT_3D('',#12651,#7993,#7994);
#6911=AXIS2_PLACEMENT_3D('',#12653,#7995,#7996);
#6912=AXIS2_PLACEMENT_3D('',#12654,#7997,#7998);
#6913=AXIS2_PLACEMENT_3D('',#12656,#7999,#8000);
#6914=AXIS2_PLACEMENT_3D('',#12658,#8002,#8003);
#6915=AXIS2_PLACEMENT_3D('',#12659,#8004,#8005);
#6916=AXIS2_PLACEMENT_3D('',#12661,#8006,#8007);
#6917=AXIS2_PLACEMENT_3D('',#12663,#8008,#8009);
#6918=AXIS2_PLACEMENT_3D('',#12664,#8010,#8011);
#6919=AXIS2_PLACEMENT_3D('',#12666,#8012,#8013);
#6920=AXIS2_PLACEMENT_3D('',#12668,#8015,#8016);
#6921=AXIS2_PLACEMENT_3D('',#12669,#8017,#8018);
#6922=AXIS2_PLACEMENT_3D('',#12671,#8019,#8020);
#6923=AXIS2_PLACEMENT_3D('',#12673,#8021,#8022);
#6924=AXIS2_PLACEMENT_3D('',#12674,#8023,#8024);
#6925=AXIS2_PLACEMENT_3D('',#12676,#8025,#8026);
#6926=AXIS2_PLACEMENT_3D('',#12678,#8028,#8029);
#6927=AXIS2_PLACEMENT_3D('',#12679,#8030,#8031);
#6928=AXIS2_PLACEMENT_3D('',#12682,#8033,#8034);
#6929=AXIS2_PLACEMENT_3D('',#12683,#8035,#8036);
#6930=AXIS2_PLACEMENT_3D('',#12686,#8038,#8039);
#6931=AXIS2_PLACEMENT_3D('',#12687,#8040,#8041);
#6932=AXIS2_PLACEMENT_3D('',#12690,#8043,#8044);
#6933=AXIS2_PLACEMENT_3D('',#12691,#8045,#8046);
#6934=AXIS2_PLACEMENT_3D('',#12694,#8048,#8049);
#6935=AXIS2_PLACEMENT_3D('',#12722,#8050,#8051);
#6936=AXIS2_PLACEMENT_3D('',#12730,#8052,#8053);
#6937=AXIS2_PLACEMENT_3D('',#12736,#8054,#8055);
#6938=AXIS2_PLACEMENT_3D('',#12739,#8056,#8057);
#6939=AXIS2_PLACEMENT_3D('',#12769,#8060,#8061);
#6940=AXIS2_PLACEMENT_3D('',#12812,#8062,#8063);
#6941=AXIS2_PLACEMENT_3D('',#12852,#8064,#8065);
#6942=AXIS2_PLACEMENT_3D('',#12863,#8066,#8067);
#6943=AXIS2_PLACEMENT_3D('',#12866,#8068,#8069);
#6944=AXIS2_PLACEMENT_3D('',#12896,#8072,#8073);
#6945=AXIS2_PLACEMENT_3D('',#12949,#8074,#8075);
#6946=AXIS2_PLACEMENT_3D('',#13089,#8077,#8078);
#6947=AXIS2_PLACEMENT_3D('',#13090,#8079,#8080);
#6948=AXIS2_PLACEMENT_3D('',#13200,#8082,#8083);
#7962=DIRECTION('axis',(0.,0.,1.));
#7963=DIRECTION('refdir',(1.,0.,0.));
#7964=DIRECTION('center_axis',(0.,0.,-1.));
#7965=DIRECTION('ref_axis',(1.,0.,0.));
#7966=DIRECTION('center_axis',(-2.77374560774598E-32,-4.07593403759339E-32,
-1.));
#7967=DIRECTION('ref_axis',(1.,0.,0.));
#7968=DIRECTION('',(0.,0.,-1.));
#7969=DIRECTION('center_axis',(-3.68477953769876E-32,1.85992248306542E-19,
1.));
#7970=DIRECTION('ref_axis',(1.,0.,0.));
#7971=DIRECTION('center_axis',(0.,0.,-1.));
#7972=DIRECTION('ref_axis',(1.,0.,0.));
#7973=DIRECTION('center_axis',(-2.77374560774598E-32,-4.07593403759339E-32,
-1.));
#7974=DIRECTION('ref_axis',(1.,0.,0.));
#7975=DIRECTION('',(0.,0.,-1.));
#7976=DIRECTION('center_axis',(-3.68477953769876E-32,1.85992248306542E-19,
1.));
#7977=DIRECTION('ref_axis',(1.,0.,0.));
#7978=DIRECTION('center_axis',(0.,0.,1.));
#7979=DIRECTION('ref_axis',(1.,0.,0.));
#7980=DIRECTION('center_axis',(0.,0.,1.));
#7981=DIRECTION('ref_axis',(1.,0.,0.));
#7982=DIRECTION('center_axis',(0.,0.,-1.));
#7983=DIRECTION('ref_axis',(1.,0.,0.));
#7984=DIRECTION('center_axis',(0.,0.,-1.));
#7985=DIRECTION('ref_axis',(1.,0.,0.));
#7986=DIRECTION('center_axis',(0.,0.,-1.));
#7987=DIRECTION('ref_axis',(1.,0.,0.));
#7988=DIRECTION('',(0.,0.,1.));
#7989=DIRECTION('center_axis',(0.,0.,1.));
#7990=DIRECTION('ref_axis',(1.,0.,0.));
#7991=DIRECTION('center_axis',(0.,0.,1.));
#7992=DIRECTION('ref_axis',(1.,0.,0.));
#7993=DIRECTION('center_axis',(0.,0.,1.));
#7994=DIRECTION('ref_axis',(1.,0.,0.));
#7995=DIRECTION('center_axis',(0.,0.,-1.));
#7996=DIRECTION('ref_axis',(1.,0.,0.));
#7997=DIRECTION('center_axis',(0.,0.,-1.));
#7998=DIRECTION('ref_axis',(1.,0.,0.));
#7999=DIRECTION('center_axis',(0.,0.,-1.));
#8000=DIRECTION('ref_axis',(1.,0.,0.));
#8001=DIRECTION('',(0.,0.,1.));
#8002=DIRECTION('center_axis',(0.,0.,1.));
#8003=DIRECTION('ref_axis',(1.,0.,0.));
#8004=DIRECTION('center_axis',(0.,0.,1.));
#8005=DIRECTION('ref_axis',(1.,0.,0.));
#8006=DIRECTION('center_axis',(0.,0.,1.));
#8007=DIRECTION('ref_axis',(1.,0.,0.));
#8008=DIRECTION('center_axis',(0.,0.,-1.));
#8009=DIRECTION('ref_axis',(1.,0.,0.));
#8010=DIRECTION('center_axis',(0.,0.,-1.));
#8011=DIRECTION('ref_axis',(1.,0.,0.));
#8012=DIRECTION('center_axis',(0.,0.,-1.));
#8013=DIRECTION('ref_axis',(1.,0.,0.));
#8014=DIRECTION('',(0.,0.,1.));
#8015=DIRECTION('center_axis',(0.,0.,1.));
#8016=DIRECTION('ref_axis',(1.,0.,0.));
#8017=DIRECTION('center_axis',(0.,0.,1.));
#8018=DIRECTION('ref_axis',(1.,0.,0.));
#8019=DIRECTION('center_axis',(0.,0.,1.));
#8020=DIRECTION('ref_axis',(1.,0.,0.));
#8021=DIRECTION('center_axis',(0.,0.,-1.));
#8022=DIRECTION('ref_axis',(1.,0.,0.));
#8023=DIRECTION('center_axis',(0.,0.,-1.));
#8024=DIRECTION('ref_axis',(1.,0.,0.));
#8025=DIRECTION('center_axis',(0.,0.,-1.));
#8026=DIRECTION('ref_axis',(1.,0.,0.));
#8027=DIRECTION('',(0.,0.,1.));
#8028=DIRECTION('center_axis',(0.,0.,1.));
#8029=DIRECTION('ref_axis',(1.,0.,0.));
#8030=DIRECTION('center_axis',(0.,0.,-1.));
#8031=DIRECTION('ref_axis',(1.,0.,0.));
#8032=DIRECTION('',(0.,0.,1.));
#8033=DIRECTION('center_axis',(-3.68477953769876E-32,1.85992248306542E-19,
1.));
#8034=DIRECTION('ref_axis',(1.,0.,0.));
#8035=DIRECTION('center_axis',(0.,0.,-1.));
#8036=DIRECTION('ref_axis',(1.,0.,0.));
#8037=DIRECTION('',(0.,0.,1.));
#8038=DIRECTION('center_axis',(-3.68477953769876E-32,1.85992248306542E-19,
1.));
#8039=DIRECTION('ref_axis',(1.,0.,0.));
#8040=DIRECTION('center_axis',(0.,0.,-1.));
#8041=DIRECTION('ref_axis',(1.,0.,0.));
#8042=DIRECTION('',(0.,0.,1.));
#8043=DIRECTION('center_axis',(-3.68477953769876E-32,1.85992248306542E-19,
1.));
#8044=DIRECTION('ref_axis',(1.,0.,0.));
#8045=DIRECTION('center_axis',(0.,0.,-1.));
#8046=DIRECTION('ref_axis',(1.,0.,0.));
#8047=DIRECTION('',(0.,0.,1.));
#8048=DIRECTION('center_axis',(-3.68477953769876E-32,1.85992248306542E-19,
1.));
#8049=DIRECTION('ref_axis',(1.,0.,0.));
#8050=DIRECTION('center_axis',(0.,1.,0.));
#8051=DIRECTION('ref_axis',(0.,0.,1.));
#8052=DIRECTION('center_axis',(0.994535543241646,-0.104398530780106,0.));
#8053=DIRECTION('ref_axis',(0.104226596285684,0.992897637377125,0.0573680949450512));
#8054=DIRECTION('center_axis',(-2.13610651414414E-33,-1.,4.07593403759339E-32));
#8055=DIRECTION('ref_axis',(0.688354575693766,0.,0.725374371012276));
#8056=DIRECTION('center_axis',(0.,1.,0.));
#8057=DIRECTION('ref_axis',(0.,0.,1.));
#8058=DIRECTION('',(2.13610651414414E-33,1.,-4.07593403759339E-32));
#8059=DIRECTION('',(-2.13610651414414E-33,-1.,4.07593403759339E-32));
#8060=DIRECTION('center_axis',(0.994535543241646,0.104398530780106,0.));
#8061=DIRECTION('ref_axis',(0.,0.,1.));
#8062=DIRECTION('center_axis',(0.979252793246429,-0.20264246079997,0.));
#8063=DIRECTION('ref_axis',(0.,0.,1.));
#8064=DIRECTION('center_axis',(0.,-1.,0.));
#8065=DIRECTION('ref_axis',(-2.77555756156289E-15,0.,1.));
#8066=DIRECTION('center_axis',(-2.13610651414429E-33,1.,-4.07593403759339E-32));
#8067=DIRECTION('ref_axis',(-0.688354575693754,0.,0.725374371012288));
#8068=DIRECTION('center_axis',(0.,-1.,0.));
#8069=DIRECTION('ref_axis',(0.,0.,1.));
#8070=DIRECTION('',(2.13610651414429E-33,-1.,4.07593403759339E-32));
#8071=DIRECTION('',(-2.13610651414429E-33,1.,-4.07593403759339E-32));
#8072=DIRECTION('center_axis',(-0.979252793246429,-0.20264246079997,-4.07695874246507E-15));
#8073=DIRECTION('ref_axis',(-4.16333634234434E-15,0.,1.));
#8074=DIRECTION('center_axis',(0.998629534754574,0.,-0.0523359562429439));
#8075=DIRECTION('ref_axis',(-0.0523359562429439,0.,-0.998629534754574));
#8076=DIRECTION('',(0.,1.,0.));
#8077=DIRECTION('center_axis',(2.77374560774598E-32,4.07593403759339E-32,
1.));
#8078=DIRECTION('ref_axis',(1.,0.,-2.77374560774598E-32));
#8079=DIRECTION('center_axis',(-0.998629534754574,0.,-0.0523359562429402));
#8080=DIRECTION('ref_axis',(-0.0523359562429402,0.,0.998629534754574));
#8081=DIRECTION('',(0.,-1.,0.));
#8082=DIRECTION('center_axis',(-3.68477953769876E-32,1.85992248306542E-19,
1.));
#8083=DIRECTION('ref_axis',(1.,0.,3.68477953769876E-32));
#12626=CARTESIAN_POINT('',(0.,0.,0.));
#12627=CARTESIAN_POINT('Origin',(2.,0.,1.));
#12628=CARTESIAN_POINT('',(1.65,4.28626379701574E-17,1.1));
#12629=CARTESIAN_POINT('Origin',(2.,0.,1.1));
#12630=CARTESIAN_POINT('',(1.65,4.28626379701574E-17,0.9));
#12631=CARTESIAN_POINT('',(1.65,4.28626379701574E-17,1.));
#12632=CARTESIAN_POINT('Origin',(2.,0.,0.9));
#12633=CARTESIAN_POINT('Origin',(10.,0.,1.));
#12634=CARTESIAN_POINT('',(9.65,4.28626379701574E-17,1.1));
#12635=CARTESIAN_POINT('Origin',(10.,0.,1.1));
#12636=CARTESIAN_POINT('',(9.65,4.28626379701574E-17,0.9));
#12637=CARTESIAN_POINT('',(9.65,4.28626379701574E-17,1.));
#12638=CARTESIAN_POINT('Origin',(10.,0.,0.9));
#12639=CARTESIAN_POINT('Origin',(9.,1.,0.7));
#12640=CARTESIAN_POINT('',(8.75,1.,0.7));
#12641=CARTESIAN_POINT('Origin',(9.,1.,0.7));
#12642=CARTESIAN_POINT('',(8.85,1.,0.7));
#12643=CARTESIAN_POINT('Origin',(9.,1.,0.7));
#12644=CARTESIAN_POINT('Origin',(9.,1.,0.7));
#12645=CARTESIAN_POINT('',(8.75,1.,0.6));
#12646=CARTESIAN_POINT('Origin',(9.,1.,0.6));
#12647=CARTESIAN_POINT('',(8.75,1.,0.7));
#12648=CARTESIAN_POINT('Origin',(9.,1.,0.6));
#12649=CARTESIAN_POINT('Origin',(3.,-1.,0.7));
#12650=CARTESIAN_POINT('',(2.75,-1.,0.7));
#12651=CARTESIAN_POINT('Origin',(3.,-1.,0.7));
#12652=CARTESIAN_POINT('',(2.85,-1.,0.7));
#12653=CARTESIAN_POINT('Origin',(3.,-1.,0.7));
#12654=CARTESIAN_POINT('Origin',(3.,-1.,0.7));
#12655=CARTESIAN_POINT('',(2.75,-1.,0.6));
#12656=CARTESIAN_POINT('Origin',(3.,-1.,0.6));
#12657=CARTESIAN_POINT('',(2.75,-1.,0.7));
#12658=CARTESIAN_POINT('Origin',(3.,-1.,0.6));
#12659=CARTESIAN_POINT('Origin',(3.,1.,0.7));
#12660=CARTESIAN_POINT('',(2.75,1.,0.7));
#12661=CARTESIAN_POINT('Origin',(3.,1.,0.7));
#12662=CARTESIAN_POINT('',(2.85,1.,0.7));
#12663=CARTESIAN_POINT('Origin',(3.,1.,0.7));
#12664=CARTESIAN_POINT('Origin',(3.,1.,0.7));
#12665=CARTESIAN_POINT('',(2.75,1.,0.6));
#12666=CARTESIAN_POINT('Origin',(3.,1.,0.6));
#12667=CARTESIAN_POINT('',(2.75,1.,0.7));
#12668=CARTESIAN_POINT('Origin',(3.,1.,0.6));
#12669=CARTESIAN_POINT('Origin',(9.,-1.,0.7));
#12670=CARTESIAN_POINT('',(8.75,-1.,0.7));
#12671=CARTESIAN_POINT('Origin',(9.,-1.,0.7));
#12672=CARTESIAN_POINT('',(8.85,-1.,0.7));
#12673=CARTESIAN_POINT('Origin',(9.,-1.,0.7));
#12674=CARTESIAN_POINT('Origin',(9.,-1.,0.7));
#12675=CARTESIAN_POINT('',(8.75,-1.,0.6));
#12676=CARTESIAN_POINT('Origin',(9.,-1.,0.6));
#12677=CARTESIAN_POINT('',(8.75,-1.,0.7));
#12678=CARTESIAN_POINT('Origin',(9.,-1.,0.6));
#12679=CARTESIAN_POINT('Origin',(9.,1.,0.9));
#12680=CARTESIAN_POINT('',(8.85,1.,0.9));
#12681=CARTESIAN_POINT('',(8.85,1.,0.9));
#12682=CARTESIAN_POINT('Origin',(9.,1.,0.9));
#12683=CARTESIAN_POINT('Origin',(3.,-1.,0.9));
#12684=CARTESIAN_POINT('',(2.85,-1.,0.9));
#12685=CARTESIAN_POINT('',(2.85,-1.,0.9));
#12686=CARTESIAN_POINT('Origin',(3.,-1.,0.9));
#12687=CARTESIAN_POINT('Origin',(3.,1.,0.9));
#12688=CARTESIAN_POINT('',(2.85,1.,0.9));
#12689=CARTESIAN_POINT('',(2.85,1.,0.9));
#12690=CARTESIAN_POINT('Origin',(3.,1.,0.9));
#12691=CARTESIAN_POINT('Origin',(9.,-1.,0.9));
#12692=CARTESIAN_POINT('',(8.85,-1.,0.9));
#12693=CARTESIAN_POINT('',(8.85,-1.,0.9));
#12694=CARTESIAN_POINT('Origin',(9.,-1.,0.9));
#12695=CARTESIAN_POINT('Ctrl Pts',(11.5038445323837,1.18103800495499,1.1));
#12696=CARTESIAN_POINT('Ctrl Pts',(11.5184054935931,1.17950950960121,1.1));
#12697=CARTESIAN_POINT('Ctrl Pts',(11.5512741038969,1.16492409601325,1.1));
#12698=CARTESIAN_POINT('Ctrl Pts',(11.5664342774515,1.13103804392606,1.1));
#12699=CARTESIAN_POINT('Ctrl Pts',(11.5664342774515,1.11151675574496,1.1));
#12700=CARTESIAN_POINT('Ctrl Pts',(11.5062520964801,1.2039732708886,1.1));
#12701=CARTESIAN_POINT('Ctrl Pts',(11.5256097704488,1.20178950015253,1.09999449529541));
#12702=CARTESIAN_POINT('Ctrl Pts',(11.5690795528293,1.18226331832779,1.09998611288251));
#12703=CARTESIAN_POINT('Ctrl Pts',(11.5893469235372,1.13750635859412,1.09999170314796));
#12704=CARTESIAN_POINT('Ctrl Pts',(11.5895723566779,1.11151675574496,1.1));
#12705=CARTESIAN_POINT('Ctrl Pts',(11.5104252001437,1.2437276609947,1.08142124563721));
#12706=CARTESIAN_POINT('Ctrl Pts',(11.5380451995806,1.2404317701584,1.0816749051734));
#12707=CARTESIAN_POINT('Ctrl Pts',(11.5998825216457,1.21232138637678,1.08202590066027));
#12708=CARTESIAN_POINT('Ctrl Pts',(11.629084458256,1.14864330516641,1.08167049691811));
#12709=CARTESIAN_POINT('Ctrl Pts',(11.629673151989,1.11151675574496,1.08129017730416));
#12710=CARTESIAN_POINT('Ctrl Pts',(11.5120790720623,1.25948300155991,1.0418569252725));
#12711=CARTESIAN_POINT('Ctrl Pts',(11.5430287132786,1.25602537746711,1.04251419789099));
#12712=CARTESIAN_POINT('Ctrl Pts',(11.6126593164611,1.22478248685392,1.04343302714342));
#12713=CARTESIAN_POINT('Ctrl Pts',(11.6451104499416,1.15305025146974,1.04249969645955));
#12714=CARTESIAN_POINT('Ctrl Pts',(11.6454164251054,1.11151675574496,1.0415166534692));
#12715=CARTESIAN_POINT('Ctrl Pts',(11.5121826600865,1.26046981594516,1.0245894475956));
#12716=CARTESIAN_POINT('Ctrl Pts',(11.5433440226796,1.25715387309455,1.02536599531596));
#12717=CARTESIAN_POINT('Ctrl Pts',(11.6137195683385,1.22584236729999,1.02645725900057));
#12718=CARTESIAN_POINT('Ctrl Pts',(11.6462638499073,1.15328744881755,1.02534682499181));
#12719=CARTESIAN_POINT('Ctrl Pts',(11.6463246402318,1.11151675574496,1.02418687649944));
#12720=CARTESIAN_POINT('',(11.5664342774515,1.11151675574496,1.1));
#12721=CARTESIAN_POINT('',(11.6463246402318,1.11151675574496,1.02418687649943));
#12722=CARTESIAN_POINT('Origin',(11.5664342774515,1.11151675574496,1.02));
#12723=CARTESIAN_POINT('',(11.5121826600865,1.26046981594516,1.0245894475956));
#12724=CARTESIAN_POINT('Ctrl Pts',(11.6463246402318,1.11151675574496,1.02418687649944));
#12725=CARTESIAN_POINT('Ctrl Pts',(11.6462638499073,1.15328744881755,1.02534682499181));
#12726=CARTESIAN_POINT('Ctrl Pts',(11.6137195683385,1.22584236729999,1.02645725900057));
#12727=CARTESIAN_POINT('Ctrl Pts',(11.5433440226796,1.25715387309455,1.02536599531596));
#12728=CARTESIAN_POINT('Ctrl Pts',(11.5121826600865,1.26046981594516,1.0245894475956));
#12729=CARTESIAN_POINT('',(11.5038445323837,1.18103800495499,1.1));
#12730=CARTESIAN_POINT('Origin',(11.5038445323837,1.18103800495499,1.02));
#12731=CARTESIAN_POINT('Ctrl Pts',(11.5038445323837,1.18103800495499,1.1));
#12732=CARTESIAN_POINT('Ctrl Pts',(11.5184054935931,1.17950950960121,1.1));
#12733=CARTESIAN_POINT('Ctrl Pts',(11.5512741038969,1.16492409601325,1.1));
#12734=CARTESIAN_POINT('Ctrl Pts',(11.5664342774515,1.13103804392606,1.1));
#12735=CARTESIAN_POINT('Ctrl Pts',(11.5664342774515,1.11151675574496,1.1));
#12736=CARTESIAN_POINT('Origin',(11.5664342774515,0.626416499322631,1.02));
#12737=CARTESIAN_POINT('',(11.5664342774515,-1.11151675574496,1.1));
#12738=CARTESIAN_POINT('',(11.6463246402318,-1.11151675574496,1.02418687649944));
#12739=CARTESIAN_POINT('Origin',(11.5664342774515,-1.11151675574496,1.02));
#12740=CARTESIAN_POINT('',(11.6463246402318,0.626416499322631,1.02418687649944));
#12741=CARTESIAN_POINT('',(11.5664342774515,0.626416499322631,1.1));
#12742=CARTESIAN_POINT('Ctrl Pts',(11.5664342774515,-1.11151675574496,1.1));
#12743=CARTESIAN_POINT('Ctrl Pts',(11.5664342774515,-1.12615772189446,1.1));
#12744=CARTESIAN_POINT('Ctrl Pts',(11.5553715698491,-1.16037133170262,1.1));
#12745=CARTESIAN_POINT('Ctrl Pts',(11.5232591473477,-1.17900001114805,1.1));
#12746=CARTESIAN_POINT('Ctrl Pts',(11.5038445323837,-1.181038004955,1.1));
#12747=CARTESIAN_POINT('Ctrl Pts',(11.5895723566779,-1.11151675574496,1.1));
#12748=CARTESIAN_POINT('Ctrl Pts',(11.5894032818222,-1.13100895790003,1.09999377736097));
#12749=CARTESIAN_POINT('Ctrl Pts',(11.5744722352599,-1.17628172883974,1.09998542409303));
#12750=CARTESIAN_POINT('Ctrl Pts',(11.5320623284624,-1.20106157657112,1.09999266039387));
#12751=CARTESIAN_POINT('Ctrl Pts',(11.5062520964801,-1.2039732708886,1.1));
#12752=CARTESIAN_POINT('Ctrl Pts',(11.6296731519891,-1.11151675574496,1.0812901773042));
#12753=CARTESIAN_POINT('Ctrl Pts',(11.6292316316889,-1.13936166783705,1.08157541701493));
#12754=CARTESIAN_POINT('Ctrl Pts',(11.6075809177182,-1.20379599023677,1.08201780166247));
#12755=CARTESIAN_POINT('Ctrl Pts',(11.547251866094,-1.23933313987557,1.08175945835248));
#12756=CARTESIAN_POINT('Ctrl Pts',(11.5104252001437,-1.24372766099475,1.08142124563725));
#12757=CARTESIAN_POINT('Ctrl Pts',(11.6454164251054,-1.11151675574496,1.0415166534692));
#12758=CARTESIAN_POINT('Ctrl Pts',(11.6451869437323,-1.14266687756763,1.04225393571265));
#12759=CARTESIAN_POINT('Ctrl Pts',(11.6213248916312,-1.21516855113593,1.04341114660737));
#12760=CARTESIAN_POINT('Ctrl Pts',(11.5533452603892,-1.25487283609854,1.04273328876464));
#12761=CARTESIAN_POINT('Ctrl Pts',(11.5120790720623,-1.25948300155991,1.0418569252725));
#12762=CARTESIAN_POINT('Ctrl Pts',(11.6463246402318,-1.11151675574496,1.02418687649944));
#12763=CARTESIAN_POINT('Ctrl Pts',(11.6462790474884,-1.14284477557865,1.02505683786953));
#12764=CARTESIAN_POINT('Ctrl Pts',(11.6225012384517,-1.21608782625165,1.02643081388051));
#12765=CARTESIAN_POINT('Ctrl Pts',(11.5537311435827,-1.25604855880689,1.02562484455705));
#12766=CARTESIAN_POINT('Ctrl Pts',(11.5121826600865,-1.26046981594517,1.0245894475956));
#12767=CARTESIAN_POINT('',(11.5038445323837,-1.181038004955,1.1));
#12768=CARTESIAN_POINT('',(11.5121826600865,-1.26046981594517,1.02458944759559));
#12769=CARTESIAN_POINT('Origin',(11.5038445323837,-1.181038004955,1.02));
#12770=CARTESIAN_POINT('Ctrl Pts',(11.5121826600865,-1.26046981594517,1.0245894475956));
#12771=CARTESIAN_POINT('Ctrl Pts',(11.5537311435827,-1.25604855880689,1.02562484455705));
#12772=CARTESIAN_POINT('Ctrl Pts',(11.6225012384517,-1.21608782625165,1.02643081388051));
#12773=CARTESIAN_POINT('Ctrl Pts',(11.6462790474884,-1.14284477557865,1.02505683786953));
#12774=CARTESIAN_POINT('Ctrl Pts',(11.6463246402318,-1.11151675574496,1.02418687649944));
#12775=CARTESIAN_POINT('Ctrl Pts',(11.5664342774515,-1.11151675574496,1.1));
#12776=CARTESIAN_POINT('Ctrl Pts',(11.5664342774515,-1.12615772189446,1.1));
#12777=CARTESIAN_POINT('Ctrl Pts',(11.5553715698491,-1.16037133170262,1.1));
#12778=CARTESIAN_POINT('Ctrl Pts',(11.5232591473477,-1.17900001114805,1.1));
#12779=CARTESIAN_POINT('Ctrl Pts',(11.5038445323837,-1.181038004955,1.1));
#12780=CARTESIAN_POINT('Ctrl Pts',(11.5038445323836,-1.181038004955,1.1));
#12781=CARTESIAN_POINT('Ctrl Pts',(9.93221394244152,-1.34601544154236,1.1));
#12782=CARTESIAN_POINT('Ctrl Pts',(7.3047417451522,-1.56119993769491,1.1));
#12783=CARTESIAN_POINT('Ctrl Pts',(3.61332606662357,-1.48882378722464,1.1));
#12784=CARTESIAN_POINT('Ctrl Pts',(1.52093096174237,-1.20661833758759,1.1));
#12785=CARTESIAN_POINT('Ctrl Pts',(0.489277774073836,-0.993132359214002,
1.1));
#12786=CARTESIAN_POINT('Ctrl Pts',(11.5062520964801,-1.2039732708886,1.1));
#12787=CARTESIAN_POINT('Ctrl Pts',(9.93427206726409,-1.36902193231914,1.10000125302342));
#12788=CARTESIAN_POINT('Ctrl Pts',(7.30574352860662,-1.58436797372637,1.10000007151586));
#12789=CARTESIAN_POINT('Ctrl Pts',(3.61166276511536,-1.51194672535434,1.09999968963322));
#12790=CARTESIAN_POINT('Ctrl Pts',(1.51730587435546,-1.22941181706429,1.10000211650891));
#12791=CARTESIAN_POINT('Ctrl Pts',(0.48461766586479,-1.01565194352286,1.1));
#12792=CARTESIAN_POINT('Ctrl Pts',(11.5104252017938,-1.24372767671385,1.08142125970198));
#12793=CARTESIAN_POINT('Ctrl Pts',(9.93784299858723,-1.40889527428921,1.08136351975694));
#12794=CARTESIAN_POINT('Ctrl Pts',(7.3074712357333,-1.62451940065184,1.08127113650551));
#12795=CARTESIAN_POINT('Ctrl Pts',(3.60878747433083,-1.55202277432172,1.08130174433006));
#12796=CARTESIAN_POINT('Ctrl Pts',(1.51101154909588,-1.26891547398152,1.08143311272106));
#12797=CARTESIAN_POINT('Ctrl Pts',(0.476539293980871,-1.05469000198791,
1.08153107638517));
#12798=CARTESIAN_POINT('Ctrl Pts',(11.5120790720622,-1.25948300155992,1.0418569252725));
#12799=CARTESIAN_POINT('Ctrl Pts',(9.93924961011084,-1.42463380902671,1.04170731179674));
#12800=CARTESIAN_POINT('Ctrl Pts',(7.30815001459807,-1.64026117966461,1.0414672686166));
#12801=CARTESIAN_POINT('Ctrl Pts',(3.60765874156876,-1.56776897899067,1.04154646081959));
#12802=CARTESIAN_POINT('Ctrl Pts',(1.50852499534242,-1.28458904017411,1.04188830921359));
#12803=CARTESIAN_POINT('Ctrl Pts',(0.473312455428654,-1.07028343020201,
1.04214267388586));
#12804=CARTESIAN_POINT('Ctrl Pts',(11.5121826600865,-1.26046981594517,1.0245894475956));
#12805=CARTESIAN_POINT('Ctrl Pts',(9.9393350416019,-1.42558521977072,1.02441268379886));
#12806=CARTESIAN_POINT('Ctrl Pts',(7.30818539134325,-1.64115782448209,1.02412850358181));
#12807=CARTESIAN_POINT('Ctrl Pts',(3.607597182252,-1.56868448653922,1.02422201615766));
#12808=CARTESIAN_POINT('Ctrl Pts',(1.50836811330665,-1.28557739750152,1.02462705425916));
#12809=CARTESIAN_POINT('Ctrl Pts',(0.473097162761967,-1.07132381406029,
1.02492790083044));
#12810=CARTESIAN_POINT('',(0.489277774073836,-0.993132359214002,1.1));
#12811=CARTESIAN_POINT('',(0.473097162761967,-1.07132381406029,1.02492790083044));
#12812=CARTESIAN_POINT('Origin',(0.489277774073836,-0.993132359214002,1.02));
#12813=CARTESIAN_POINT('Ctrl Pts',(0.473097162761967,-1.07132381406029,
1.02492790083044));
#12814=CARTESIAN_POINT('Ctrl Pts',(1.50836811330665,-1.28557739750152,1.02462705425916));
#12815=CARTESIAN_POINT('Ctrl Pts',(3.607597182252,-1.56868448653922,1.02422201615766));
#12816=CARTESIAN_POINT('Ctrl Pts',(7.30818539134325,-1.64115782448209,1.02412850358181));
#12817=CARTESIAN_POINT('Ctrl Pts',(9.9393350416019,-1.42558521977072,1.02441268379886));
#12818=CARTESIAN_POINT('Ctrl Pts',(11.5121826600865,-1.26046981594517,1.0245894475956));
#12819=CARTESIAN_POINT('Ctrl Pts',(11.5038445323836,-1.181038004955,1.1));
#12820=CARTESIAN_POINT('Ctrl Pts',(9.93221394244152,-1.34601544154236,1.1));
#12821=CARTESIAN_POINT('Ctrl Pts',(7.3047417451522,-1.56119993769491,1.1));
#12822=CARTESIAN_POINT('Ctrl Pts',(3.61332606662357,-1.48882378722464,1.1));
#12823=CARTESIAN_POINT('Ctrl Pts',(1.52093096174237,-1.20661833758759,1.1));
#12824=CARTESIAN_POINT('Ctrl Pts',(0.489277774073836,-0.993132359214002,
1.1));
#12825=CARTESIAN_POINT('Ctrl Pts',(0.489277774073836,-0.993132359214003,
1.1));
#12826=CARTESIAN_POINT('Ctrl Pts',(0.47591459116406,-0.990367038259462,
1.1));
#12827=CARTESIAN_POINT('Ctrl Pts',(0.446638556739065,-0.974524902741032,
1.1));
#12828=CARTESIAN_POINT('Ctrl Pts',(0.433565722548535,-0.942876078073176,
1.1));
#12829=CARTESIAN_POINT('Ctrl Pts',(0.433565722548535,-0.924681003894255,
1.1));
#12830=CARTESIAN_POINT('Ctrl Pts',(0.48461766586479,-1.01565194352286,1.1));
#12831=CARTESIAN_POINT('Ctrl Pts',(0.466871946563175,-1.01185427439077,
1.09999555360656));
#12832=CARTESIAN_POINT('Ctrl Pts',(0.428148998320346,-0.990723083341879,
1.0999884677795));
#12833=CARTESIAN_POINT('Ctrl Pts',(0.410637366989639,-0.948905017863894,
1.09999228132016));
#12834=CARTESIAN_POINT('Ctrl Pts',(0.410427643322096,-0.924681003894255,
1.1));
#12835=CARTESIAN_POINT('Ctrl Pts',(0.47653584926364,-1.05470664829667,1.08154627613271));
#12836=CARTESIAN_POINT('Ctrl Pts',(0.451238756159369,-1.04914377880765,
1.08175207965746));
#12837=CARTESIAN_POINT('Ctrl Pts',(0.396142217510869,-1.01881823177681,
1.08201099971769));
#12838=CARTESIAN_POINT('Ctrl Pts',(0.370857020273576,-0.959285462196374,
1.08165947596025));
#12839=CARTESIAN_POINT('Ctrl Pts',(0.370309350093454,-0.924681003894255,
1.0813056591965));
#12840=CARTESIAN_POINT('Ctrl Pts',(0.473312455428654,-1.07028343020201,
1.04214267388586));
#12841=CARTESIAN_POINT('Ctrl Pts',(0.444929265438756,-1.064235408557,1.04267704697817));
#12842=CARTESIAN_POINT('Ctrl Pts',(0.382898223041383,-1.03040761468413,
1.04335444671884));
#12843=CARTESIAN_POINT('Ctrl Pts',(0.354868227955524,-0.963393056722486,
1.04243119239046));
#12844=CARTESIAN_POINT('Ctrl Pts',(0.354583574894625,-0.924681003894255,
1.0415166534692));
#12845=CARTESIAN_POINT('Ctrl Pts',(0.473097162761967,-1.07132381406029,
1.02492790083044));
#12846=CARTESIAN_POINT('Ctrl Pts',(0.444494893732137,-1.06536514830602,
1.02555992378854));
#12847=CARTESIAN_POINT('Ctrl Pts',(0.381802689524125,-1.03137574421946,
1.02636429433614));
#12848=CARTESIAN_POINT('Ctrl Pts',(0.353731913874551,-0.963614141904928,
1.02526599313355));
#12849=CARTESIAN_POINT('Ctrl Pts',(0.35367535976817,-0.924681003894255,
1.02418687649944));
#12850=CARTESIAN_POINT('',(0.433565722548535,-0.924681003894255,1.1));
#12851=CARTESIAN_POINT('',(0.35367535976817,-0.924681003894255,1.02418687649944));
#12852=CARTESIAN_POINT('Origin',(0.433565722548536,-0.924681003894255,1.02));
#12853=CARTESIAN_POINT('Ctrl Pts',(0.35367535976817,-0.924681003894255,
1.02418687649944));
#12854=CARTESIAN_POINT('Ctrl Pts',(0.353731913874551,-0.963614141904928,
1.02526599313355));
#12855=CARTESIAN_POINT('Ctrl Pts',(0.381802689524125,-1.03137574421946,
1.02636429433614));
#12856=CARTESIAN_POINT('Ctrl Pts',(0.444494893732137,-1.06536514830602,
1.02555992378854));
#12857=CARTESIAN_POINT('Ctrl Pts',(0.473097162761967,-1.07132381406029,
1.02492790083044));
#12858=CARTESIAN_POINT('Ctrl Pts',(0.489277774073836,-0.993132359214003,
1.1));
#12859=CARTESIAN_POINT('Ctrl Pts',(0.47591459116406,-0.990367038259462,
1.1));
#12860=CARTESIAN_POINT('Ctrl Pts',(0.446638556739065,-0.974524902741032,
1.1));
#12861=CARTESIAN_POINT('Ctrl Pts',(0.433565722548535,-0.942876078073176,
1.1));
#12862=CARTESIAN_POINT('Ctrl Pts',(0.433565722548535,-0.924681003894255,
1.1));
#12863=CARTESIAN_POINT('Origin',(0.433565722548536,-0.526416499322631,1.02));
#12864=CARTESIAN_POINT('',(0.433565722548536,0.924681003894255,1.1));
#12865=CARTESIAN_POINT('',(0.35367535976817,0.924681003894255,1.02418687649944));
#12866=CARTESIAN_POINT('Origin',(0.433565722548536,0.924681003894255,1.02));
#12867=CARTESIAN_POINT('',(0.35367535976817,-0.526416499322631,1.02418687649944));
#12868=CARTESIAN_POINT('',(0.433565722548536,-0.526416499322631,1.1));
#12869=CARTESIAN_POINT('Ctrl Pts',(0.433565722548535,0.924681003894255,
1.1));
#12870=CARTESIAN_POINT('Ctrl Pts',(0.433565722548535,0.94287607801605,1.1));
#12871=CARTESIAN_POINT('Ctrl Pts',(0.44664012289244,0.97452669098104,1.1));
#12872=CARTESIAN_POINT('Ctrl Pts',(0.475914591206016,0.990367038268144,
1.1));
#12873=CARTESIAN_POINT('Ctrl Pts',(0.489277774073836,0.993132359214003,
1.1));
#12874=CARTESIAN_POINT('Ctrl Pts',(0.410427643322096,0.924681003894255,
1.1));
#12875=CARTESIAN_POINT('Ctrl Pts',(0.410637366988981,0.948905017787839,
1.09999228132018));
#12876=CARTESIAN_POINT('Ctrl Pts',(0.428151078432557,0.99072545440496,1.09998846767325));
#12877=CARTESIAN_POINT('Ctrl Pts',(0.466871946618891,1.01185427440269,1.09999555360657));
#12878=CARTESIAN_POINT('Ctrl Pts',(0.48461766586479,1.01565194352286,1.1));
#12879=CARTESIAN_POINT('Ctrl Pts',(0.370309350093454,0.924681003894255,
1.0813056591965));
#12880=CARTESIAN_POINT('Ctrl Pts',(0.370857020271857,0.959285462087728,
1.08165947595914));
#12881=CARTESIAN_POINT('Ctrl Pts',(0.396145183504025,1.01882160767722,1.08201100382378));
#12882=CARTESIAN_POINT('Ctrl Pts',(0.451238756238795,1.04914377882512,1.08175207965681));
#12883=CARTESIAN_POINT('Ctrl Pts',(0.47653584926364,1.05470664829667,1.08154627613271));
#12884=CARTESIAN_POINT('Ctrl Pts',(0.354583574894625,0.924681003894255,
1.0415166534692));
#12885=CARTESIAN_POINT('Ctrl Pts',(0.35486822795463,0.963393056600943,1.04243119238759));
#12886=CARTESIAN_POINT('Ctrl Pts',(0.382901552879886,1.03041141096935,1.04335445746542));
#12887=CARTESIAN_POINT('Ctrl Pts',(0.444929265527871,1.06423540857599,1.04267704697649));
#12888=CARTESIAN_POINT('Ctrl Pts',(0.473312455428654,1.07028343020201,1.04214267388586));
#12889=CARTESIAN_POINT('Ctrl Pts',(0.35367535976817,0.924681003894255,1.02418687649944));
#12890=CARTESIAN_POINT('Ctrl Pts',(0.353731913874373,0.963614141782691,
1.02526599313016));
#12891=CARTESIAN_POINT('Ctrl Pts',(0.381806046235973,1.03137957549636,1.02636430709951));
#12892=CARTESIAN_POINT('Ctrl Pts',(0.44449489382194,1.06536514832473,1.02555992378656));
#12893=CARTESIAN_POINT('Ctrl Pts',(0.473097162761967,1.07132381406029,1.02492790083044));
#12894=CARTESIAN_POINT('',(0.489277774073836,0.993132359214003,1.1));
#12895=CARTESIAN_POINT('',(0.473097162761967,1.07132381406029,1.02492790083044));
#12896=CARTESIAN_POINT('Origin',(0.489277774073836,0.993132359214003,1.02));
#12897=CARTESIAN_POINT('Ctrl Pts',(0.473097162761967,1.07132381406029,1.02492790083044));
#12898=CARTESIAN_POINT('Ctrl Pts',(0.44449489382194,1.06536514832473,1.02555992378656));
#12899=CARTESIAN_POINT('Ctrl Pts',(0.381806046235973,1.03137957549636,1.02636430709951));
#12900=CARTESIAN_POINT('Ctrl Pts',(0.353731913874373,0.963614141782691,
1.02526599313016));
#12901=CARTESIAN_POINT('Ctrl Pts',(0.35367535976817,0.924681003894255,1.02418687649944));
#12902=CARTESIAN_POINT('Ctrl Pts',(0.433565722548535,0.924681003894255,
1.1));
#12903=CARTESIAN_POINT('Ctrl Pts',(0.433565722548535,0.94287607801605,1.1));
#12904=CARTESIAN_POINT('Ctrl Pts',(0.44664012289244,0.97452669098104,1.1));
#12905=CARTESIAN_POINT('Ctrl Pts',(0.475914591206016,0.990367038268144,
1.1));
#12906=CARTESIAN_POINT('Ctrl Pts',(0.489277774073836,0.993132359214003,
1.1));
#12907=CARTESIAN_POINT('Ctrl Pts',(0.489277774073836,0.993132359214003,
1.1));
#12908=CARTESIAN_POINT('Ctrl Pts',(1.52092917355268,1.20661796754713,1.1));
#12909=CARTESIAN_POINT('Ctrl Pts',(3.61335021200387,1.48882484395407,1.1));
#12910=CARTESIAN_POINT('Ctrl Pts',(7.30471495328446,1.56119985233321,1.1));
#12911=CARTESIAN_POINT('Ctrl Pts',(9.93221666658724,1.34601515558293,1.1));
#12912=CARTESIAN_POINT('Ctrl Pts',(11.5038445323836,1.18103800495499,1.1));
#12913=CARTESIAN_POINT('Ctrl Pts',(0.48461766586479,1.01565194352286,1.1));
#12914=CARTESIAN_POINT('Ctrl Pts',(1.51730408437175,1.22941144654908,1.10000211650524));
#12915=CARTESIAN_POINT('Ctrl Pts',(3.61168692820091,1.5119477834436,1.09999968963693));
#12916=CARTESIAN_POINT('Ctrl Pts',(7.30571671988008,1.58436788793099,1.10000007151498));
#12917=CARTESIAN_POINT('Ctrl Pts',(9.9342747920155,1.36902164623626,1.10000125302125));
#12918=CARTESIAN_POINT('Ctrl Pts',(11.5062520964801,1.2039732708886,1.1));
#12919=CARTESIAN_POINT('Ctrl Pts',(0.476539293980872,1.05469000198791,1.08153107638517));
#12920=CARTESIAN_POINT('Ctrl Pts',(1.51100975601983,1.26891510265927,1.08143311289086));
#12921=CARTESIAN_POINT('Ctrl Pts',(3.60881166804804,1.5520238347382,1.08130174382265));
#12922=CARTESIAN_POINT('Ctrl Pts',(7.30744439783659,1.62451931411139,1.08127113658549));
#12923=CARTESIAN_POINT('Ctrl Pts',(9.9378457243824,1.40889498800017,1.08136351985702));
#12924=CARTESIAN_POINT('Ctrl Pts',(11.5104252017938,1.24372767671385,1.08142125970198));
#12925=CARTESIAN_POINT('Ctrl Pts',(0.473312455428654,1.07028343020201,1.04214267388586));
#12926=CARTESIAN_POINT('Ctrl Pts',(1.50852320098322,1.28458866871296,1.04188830965449));
#12927=CARTESIAN_POINT('Ctrl Pts',(3.60768294746331,1.5677700397583,1.04154645950336));
#12928=CARTESIAN_POINT('Ctrl Pts',(7.30812316513016,1.64026109291585,1.04146726882447));
#12929=CARTESIAN_POINT('Ctrl Pts',(9.93925233633459,1.42463352276678,1.04170731205607));
#12930=CARTESIAN_POINT('Ctrl Pts',(11.5120790720622,1.25948300155991,1.0418569252725));
#12931=CARTESIAN_POINT('Ctrl Pts',(0.473097162761967,1.07132381406029,1.02492790083044));
#12932=CARTESIAN_POINT('Ctrl Pts',(1.50836631884621,1.28557702613055,1.02462705478063));
#12933=CARTESIAN_POINT('Ctrl Pts',(3.60762138890097,1.56868554702656,1.02422201460129));
#12934=CARTESIAN_POINT('Ctrl Pts',(7.30815854116978,1.64115773776738,1.02412850382783));
#12935=CARTESIAN_POINT('Ctrl Pts',(9.93933776785713,1.42558493357216,1.02441268410525));
#12936=CARTESIAN_POINT('Ctrl Pts',(11.5121826600865,1.26046981594517,1.0245894475956));
#12937=CARTESIAN_POINT('Ctrl Pts',(11.5121826600865,1.26046981594517,1.0245894475956));
#12938=CARTESIAN_POINT('Ctrl Pts',(9.93933776785713,1.42558493357216,1.02441268410525));
#12939=CARTESIAN_POINT('Ctrl Pts',(7.30815854116978,1.64115773776738,1.02412850382783));
#12940=CARTESIAN_POINT('Ctrl Pts',(3.60762138890097,1.56868554702656,1.02422201460129));
#12941=CARTESIAN_POINT('Ctrl Pts',(1.50836631884621,1.28557702613055,1.02462705478063));
#12942=CARTESIAN_POINT('Ctrl Pts',(0.473097162761967,1.07132381406029,1.02492790083044));
#12943=CARTESIAN_POINT('Ctrl Pts',(0.489277774073836,0.993132359214003,
1.1));
#12944=CARTESIAN_POINT('Ctrl Pts',(1.52092917355268,1.20661796754713,1.1));
#12945=CARTESIAN_POINT('Ctrl Pts',(3.61335021200387,1.48882484395407,1.1));
#12946=CARTESIAN_POINT('Ctrl Pts',(7.30471495328446,1.56119985233321,1.1));
#12947=CARTESIAN_POINT('Ctrl Pts',(9.93221666658724,1.34601515558293,1.1));
#12948=CARTESIAN_POINT('Ctrl Pts',(11.5038445323836,1.18103800495499,1.1));
#12949=CARTESIAN_POINT('Origin',(0.347167001354737,-1.05283299864526,0.9));
#12950=CARTESIAN_POINT('',(0.347167001354737,0.931160914046453,0.9));
#12951=CARTESIAN_POINT('Ctrl Pts',(0.347167001354737,0.931160914046453,
0.9));
#12952=CARTESIAN_POINT('Ctrl Pts',(0.34933645413337,0.929000934518636,0.941395625006663));
#12953=CARTESIAN_POINT('Ctrl Pts',(0.351505906937822,0.926840964458487,
0.982791250505987));
#12954=CARTESIAN_POINT('Ctrl Pts',(0.35367535976817,0.924681003894255,1.02418687649944));
#12955=CARTESIAN_POINT('',(0.347167001354737,-0.931160914046453,0.9));
#12956=CARTESIAN_POINT('',(0.347167001354737,-1.05283299864526,0.9));
#12957=CARTESIAN_POINT('Ctrl Pts',(0.35367535976817,-0.924681003894255,
1.02418687649944));
#12958=CARTESIAN_POINT('Ctrl Pts',(0.351505906937822,-0.926840964458487,
0.982791250505987));
#12959=CARTESIAN_POINT('Ctrl Pts',(0.34933645413337,-0.929000934518636,
0.941395625006663));
#12960=CARTESIAN_POINT('Ctrl Pts',(0.347167001354737,-0.931160914046453,
0.9));
#12961=CARTESIAN_POINT('Ctrl Pts',(0.346994979645257,0.93133218461645,0.89671763024815));
#12962=CARTESIAN_POINT('Ctrl Pts',(0.349221772992334,0.929115114391563,
0.939207378479044));
#12963=CARTESIAN_POINT('Ctrl Pts',(0.35144856636661,0.926898054140648,0.981697127228945));
#12964=CARTESIAN_POINT('Ctrl Pts',(0.35367535976817,0.924681003894255,1.02418687649944));
#12965=CARTESIAN_POINT('Ctrl Pts',(0.347101141748081,0.970260862175626,
0.898743323843195));
#12966=CARTESIAN_POINT('Ctrl Pts',(0.349327989245423,0.968041585482289,
0.94123294798136));
#12967=CARTESIAN_POINT('Ctrl Pts',(0.35155465541633,0.96582239703375,0.983722586263841));
#12968=CARTESIAN_POINT('Ctrl Pts',(0.353781503060223,0.96360313540272,1.02621221116359));
#12969=CARTESIAN_POINT('Ctrl Pts',(0.375231247034764,1.03797686888013,0.90080243726586));
#12970=CARTESIAN_POINT('Ctrl Pts',(0.377454726329371,1.03575393200526,0.943292036336267));
#12971=CARTESIAN_POINT('Ctrl Pts',(0.379678256934949,1.03353096064141,0.985781630873016));
#12972=CARTESIAN_POINT('Ctrl Pts',(0.381901729528225,1.03130803054038,1.02827123060239));
#12973=CARTESIAN_POINT('Ctrl Pts',(0.437891832981715,1.07196344732884,0.899291918906528));
#12974=CARTESIAN_POINT('Ctrl Pts',(0.440109459023804,1.06974216787274,0.941781905864285));
#12975=CARTESIAN_POINT('Ctrl Pts',(0.442327107866739,1.06752094195844,0.984271894420663));
#12976=CARTESIAN_POINT('Ctrl Pts',(0.44454471435444,1.06529967134173,1.02676188280081));
#12977=CARTESIAN_POINT('Ctrl Pts',(0.466484255634356,1.07794817238022,0.898105730168711));
#12978=CARTESIAN_POINT('Ctrl Pts',(0.46869984010673,1.07572875745303,0.940595920481163));
#12979=CARTESIAN_POINT('Ctrl Pts',(0.470915412358444,1.07350934859911,0.983086111716909));
#12980=CARTESIAN_POINT('Ctrl Pts',(0.473130972350001,1.07128994583173,1.02557630387858));
#12981=CARTESIAN_POINT('',(0.466583029361855,1.07784922788182,0.9));
#12982=CARTESIAN_POINT('Ctrl Pts',(0.473097162761967,1.07132381406029,1.02492790083044));
#12983=CARTESIAN_POINT('Ctrl Pts',(0.470925796725269,1.07349894615889,0.983285266331776));
#12984=CARTESIAN_POINT('Ctrl Pts',(0.468754418912838,1.07567408410356,0.941642632722456));
#12985=CARTESIAN_POINT('Ctrl Pts',(0.466583029361855,1.07784922788182,0.9));
#12986=CARTESIAN_POINT('Ctrl Pts',(0.466583029361856,1.07784922788182,0.9));
#12987=CARTESIAN_POINT('Ctrl Pts',(0.45605169130101,1.07567238924625,0.899999999995368));
#12988=CARTESIAN_POINT('Ctrl Pts',(0.445810809951917,1.07234818111891,0.899998625774342));
#12989=CARTESIAN_POINT('Ctrl Pts',(0.436024610942277,1.06798890472683,0.899998407511246));
#12990=CARTESIAN_POINT('Ctrl Pts',(0.42804650025127,1.0644350438709,0.899998229574221));
#12991=CARTESIAN_POINT('Ctrl Pts',(0.420370119207661,1.06019193848671,0.899998775177391));
#12992=CARTESIAN_POINT('Ctrl Pts',(0.413095080427888,1.05529723033767,0.89999964722522));
#12993=CARTESIAN_POINT('Ctrl Pts',(0.404948343152914,1.04981603600524,0.900000623762221));
#12994=CARTESIAN_POINT('Ctrl Pts',(0.3973835293994,1.04357129238854,0.900002055204145));
#12995=CARTESIAN_POINT('Ctrl Pts',(0.390528747317286,1.03663323920468,0.900000884971142));
#12996=CARTESIAN_POINT('Ctrl Pts',(0.38377850537204,1.02980099609921,0.899999732584995));
#12997=CARTESIAN_POINT('Ctrl Pts',(0.377716121663402,1.02229558340178,0.899996048870533));
#12998=CARTESIAN_POINT('Ctrl Pts',(0.372394770625083,1.01423711207676,0.899993306941804));
#12999=CARTESIAN_POINT('Ctrl Pts',(0.366459905306112,1.00524955578769,0.899990248888012));
#13000=CARTESIAN_POINT('Ctrl Pts',(0.361501411166698,0.995658501454654,
0.8999884459165));
#13001=CARTESIAN_POINT('Ctrl Pts',(0.35758177265536,0.985639755107121,0.899989063766683));
#13002=CARTESIAN_POINT('Ctrl Pts',(0.356156017388132,0.981995469968403,
0.8999892885076));
#13003=CARTESIAN_POINT('Ctrl Pts',(0.354868143601992,0.978294337124559,
0.899989797558581));
#13004=CARTESIAN_POINT('Ctrl Pts',(0.353722739999278,0.97454418014098,0.899990530873797));
#13005=CARTESIAN_POINT('Ctrl Pts',(0.350595356382139,0.964304837882626,
0.899992533100777));
#13006=CARTESIAN_POINT('Ctrl Pts',(0.348551371116014,0.953782216732967,
0.899996407005639));
#13007=CARTESIAN_POINT('Ctrl Pts',(0.347666342074759,0.943140644221274,
0.899998614621972));
#13008=CARTESIAN_POINT('Ctrl Pts',(0.347335396628921,0.939161362417926,
0.899999440132251));
#13009=CARTESIAN_POINT('Ctrl Pts',(0.347167001797138,0.935165318330998,
0.899999999966431));
#13010=CARTESIAN_POINT('Ctrl Pts',(0.347167001354737,0.931160914046453,
0.9));
#13011=CARTESIAN_POINT('Ctrl Pts',(0.466583029361855,1.07784922788182,0.9));
#13012=CARTESIAN_POINT('Ctrl Pts',(0.468719324182819,1.07566682993082,0.941642633610146));
#13013=CARTESIAN_POINT('Ctrl Pts',(0.470855619003782,1.07348443197981,0.983285267220292));
#13014=CARTESIAN_POINT('Ctrl Pts',(0.472991913824746,1.07130203402881,1.02492790083044));
#13015=CARTESIAN_POINT('Ctrl Pts',(4.1506201585889,1.83934349355009,0.9));
#13016=CARTESIAN_POINT('Ctrl Pts',(4.15133415151554,1.83716109559909,0.941642633610146));
#13017=CARTESIAN_POINT('Ctrl Pts',(4.15204814444219,1.83497869764808,0.983285267220293));
#13018=CARTESIAN_POINT('Ctrl Pts',(4.15276213736883,1.83279629969708,1.02492790083044));
#13019=CARTESIAN_POINT('Ctrl Pts',(7.83465728781595,1.65326443611903,0.9));
#13020=CARTESIAN_POINT('Ctrl Pts',(7.83394897884827,1.65108203816803,0.941642633610146));
#13021=CARTESIAN_POINT('Ctrl Pts',(7.83324066988059,1.64889964021702,0.983285267220292));
#13022=CARTESIAN_POINT('Ctrl Pts',(7.83253236091292,1.64671724226602,1.02492790083044));
#13023=CARTESIAN_POINT('Ctrl Pts',(11.518694417043,1.26698486563531,0.9));
#13024=CARTESIAN_POINT('Ctrl Pts',(11.516563806181,1.26480246768431,0.941642633610146));
#13025=CARTESIAN_POINT('Ctrl Pts',(11.514433195319,1.2626200697333,0.983285267220292));
#13026=CARTESIAN_POINT('Ctrl Pts',(11.512302584457,1.2604376717823,1.02492790083044));
#13027=CARTESIAN_POINT('',(11.518694417043,1.26698486563531,0.9));
#13028=CARTESIAN_POINT('Ctrl Pts',(11.518694417043,1.26698486563531,0.9));
#13029=CARTESIAN_POINT('Ctrl Pts',(11.5165238247878,1.26481317761477,0.941529815291285));
#13030=CARTESIAN_POINT('Ctrl Pts',(11.5143532391283,1.26264149437998,0.983059631155884));
#13031=CARTESIAN_POINT('Ctrl Pts',(11.5121826600865,1.26046981594516,1.0245894475956));
#13032=CARTESIAN_POINT('Ctrl Pts',(0.466583029361855,1.07784922788182,0.9));
#13033=CARTESIAN_POINT('Ctrl Pts',(4.1506201585889,1.83934349355009,0.9));
#13034=CARTESIAN_POINT('Ctrl Pts',(7.83465728781595,1.65326443611903,0.9));
#13035=CARTESIAN_POINT('Ctrl Pts',(11.518694417043,1.26698486563531,0.9));
#13036=CARTESIAN_POINT('Ctrl Pts',(11.5188237574534,1.26711427133763,0.897525337604991));
#13037=CARTESIAN_POINT('Ctrl Pts',(11.5166039145442,1.26489330787379,0.939997457644392));
#13038=CARTESIAN_POINT('Ctrl Pts',(11.5143840785328,1.26267234941507,0.982469578283382));
#13039=CARTESIAN_POINT('Ctrl Pts',(11.512164249443,1.26045139597664,1.02494169952389));
#13040=CARTESIAN_POINT('Ctrl Pts',(11.560356924166,1.2626472646828,0.899468475190601));
#13041=CARTESIAN_POINT('Ctrl Pts',(11.5581357517162,1.26042470505353,0.941940442504879));
#13042=CARTESIAN_POINT('Ctrl Pts',(11.5559146107476,1.25820228015812,0.984412418590584));
#13043=CARTESIAN_POINT('Ctrl Pts',(11.5536934488601,1.25597972716877,1.02688438676053));
#13044=CARTESIAN_POINT('Ctrl Pts',(11.6290545561482,1.22266466287338,0.9009785794625));
#13045=CARTESIAN_POINT('Ctrl Pts',(11.6268300646776,1.22044146949289,0.943450343593379));
#13046=CARTESIAN_POINT('Ctrl Pts',(11.6246055668724,1.21821824717544,0.985922105839347));
#13047=CARTESIAN_POINT('Ctrl Pts',(11.6223810783988,1.21599505938238,1.02839387038768));
#13048=CARTESIAN_POINT('Ctrl Pts',(11.652916631058,1.14949843694546,0.898404198500408));
#13049=CARTESIAN_POINT('Ctrl Pts',(11.6506907663731,1.14727726203421,0.940876003223652));
#13050=CARTESIAN_POINT('Ctrl Pts',(11.6484649368037,1.14505607393729,0.9833478090785));
#13051=CARTESIAN_POINT('Ctrl Pts',(11.6462390720682,1.14283490928962,1.02581961432614));
#13052=CARTESIAN_POINT('Ctrl Pts',(11.6530022067803,1.11817769023529,0.896771316447588));
#13053=CARTESIAN_POINT('Ctrl Pts',(11.6507763512808,1.11595737261641,0.939243169479033));
#13054=CARTESIAN_POINT('Ctrl Pts',(11.6485504957647,1.11373706111287,0.981715022829298));
#13055=CARTESIAN_POINT('Ctrl Pts',(11.6463246402318,1.11151675574496,1.02418687649944));
#13056=CARTESIAN_POINT('',(11.6528329986453,1.11800890309831,0.9));
#13057=CARTESIAN_POINT('Ctrl Pts',(11.6463246402318,1.11151675574496,1.02418687649944));
#13058=CARTESIAN_POINT('Ctrl Pts',(11.6484940930522,1.11368079904038,0.982791250696082));
#13059=CARTESIAN_POINT('Ctrl Pts',(11.6506635458567,1.11584484816443,0.941395625196594));
#13060=CARTESIAN_POINT('Ctrl Pts',(11.6528329986453,1.11800890309831,0.9));
#13061=CARTESIAN_POINT('Ctrl Pts',(11.6528329986453,1.11800890309831,0.9));
#13062=CARTESIAN_POINT('Ctrl Pts',(11.6528329983633,1.12876627611802,0.899999999993021));
#13063=CARTESIAN_POINT('Ctrl Pts',(11.6516446702457,1.13947128553817,0.899998527904116));
#13064=CARTESIAN_POINT('Ctrl Pts',(11.6493511293179,1.14994150848088,0.899998119066462));
#13065=CARTESIAN_POINT('Ctrl Pts',(11.6474764306251,1.15849967852608,0.89999778488999));
#13066=CARTESIAN_POINT('Ctrl Pts',(11.6448621032167,1.16690170462481,0.899998134702192));
#13067=CARTESIAN_POINT('Ctrl Pts',(11.6415284502961,1.17504213011111,0.899998933310541));
#13068=CARTESIAN_POINT('Ctrl Pts',(11.6374537398456,1.18499213918264,0.899999909446287));
#13069=CARTESIAN_POINT('Ctrl Pts',(11.6323486952005,1.19444663470912,0.900001674548864));
#13070=CARTESIAN_POINT('Ctrl Pts',(11.6262733681268,1.20322237541324,0.900000560254235));
#13071=CARTESIAN_POINT('Ctrl Pts',(11.6256011619285,1.20419336960417,0.900000436962806));
#13072=CARTESIAN_POINT('Ctrl Pts',(11.6249170295004,1.20515603220147,0.900000274771288));
#13073=CARTESIAN_POINT('Ctrl Pts',(11.6242210175348,1.20611009565643,0.900000065883751));
#13074=CARTESIAN_POINT('Ctrl Pts',(11.6197944794931,1.21217780481426,0.899998737388448));
#13075=CARTESIAN_POINT('Ctrl Pts',(11.6148881172219,1.21789846943619,0.899995595976687));
#13076=CARTESIAN_POINT('Ctrl Pts',(11.6095544776251,1.22323873890669,0.899992615091414));
#13077=CARTESIAN_POINT('Ctrl Pts',(11.601940589012,1.23086209181126,0.899988359811689));
#13078=CARTESIAN_POINT('Ctrl Pts',(11.5935341028624,1.23763544449334,0.899984652834703));
#13079=CARTESIAN_POINT('Ctrl Pts',(11.584505756877,1.24347857204465,0.899983891616646));
#13080=CARTESIAN_POINT('Ctrl Pts',(11.5791642013329,1.24693561616068,0.899983441247493));
#13081=CARTESIAN_POINT('Ctrl Pts',(11.5736041411459,1.25006639925598,0.89998394495257));
#13082=CARTESIAN_POINT('Ctrl Pts',(11.5678562300951,1.25284717822614,0.899985279956182));
#13083=CARTESIAN_POINT('Ctrl Pts',(11.5582100984591,1.25751387535486,0.899987520356298));
#13084=CARTESIAN_POINT('Ctrl Pts',(11.548125859505,1.26115381593413,0.899992245475585));
#13085=CARTESIAN_POINT('Ctrl Pts',(11.5377575652696,1.26367454383615,0.899995957332528));
#13086=CARTESIAN_POINT('Ctrl Pts',(11.5314967650479,1.26519666246525,0.899998198703601));
#13087=CARTESIAN_POINT('Ctrl Pts',(11.5251318445822,1.26630988651457,0.89999999997641));
#13088=CARTESIAN_POINT('Ctrl Pts',(11.518694417043,1.26698486563531,0.900000000000001));
#13089=CARTESIAN_POINT('Origin',(6.0828528088686,0.,1.1));
#13090=CARTESIAN_POINT('Origin',(11.6528329986453,1.25283299864526,0.9));
#13091=CARTESIAN_POINT('',(11.6528329986453,-1.11800890309831,0.9));
#13092=CARTESIAN_POINT('Ctrl Pts',(11.6528329986453,-1.11800890309831,0.9));
#13093=CARTESIAN_POINT('Ctrl Pts',(11.6506635458567,-1.11584484816443,0.941395625196595));
#13094=CARTESIAN_POINT('Ctrl Pts',(11.6484940930522,-1.11368079904038,0.98279125069608));
#13095=CARTESIAN_POINT('Ctrl Pts',(11.6463246402318,-1.11151675574497,1.02418687649944));
#13096=CARTESIAN_POINT('',(11.6528329986453,1.25283299864526,0.9));
#13097=CARTESIAN_POINT('Ctrl Pts',(0.466487690105381,-1.07794473197144,
0.898171596006697));
#13098=CARTESIAN_POINT('Ctrl Pts',(0.468702129741454,-1.07572646385346,
0.940639831040774));
#13099=CARTESIAN_POINT('Ctrl Pts',(0.470916557169473,-1.07350820180247,
0.983108066997194));
#13100=CARTESIAN_POINT('Ctrl Pts',(0.473130972350001,-1.07128994583173,
1.02557630387858));
#13101=CARTESIAN_POINT('Ctrl Pts',(0.428364464143914,-1.0699650947497,0.899753180570758));
#13102=CARTESIAN_POINT('Ctrl Pts',(0.430581658228805,-1.06774429850715,
0.942221140547455));
#13103=CARTESIAN_POINT('Ctrl Pts',(0.432798785432897,-1.06552370176641,
0.98468911452651));
#13104=CARTESIAN_POINT('Ctrl Pts',(0.435015961689253,-1.0633029131784,1.02715707577488));
#13105=CARTESIAN_POINT('Ctrl Pts',(0.367703220512368,-1.02873213740117,
0.900780809445176));
#13106=CARTESIAN_POINT('Ctrl Pts',(0.369926480243704,-1.02651076835199,
0.943248428164859));
#13107=CARTESIAN_POINT('Ctrl Pts',(0.372149767842394,-1.02428934262989,
0.985716042409561));
#13108=CARTESIAN_POINT('Ctrl Pts',(0.374373022752712,-1.02206798136513,
1.0281836617465));
#13109=CARTESIAN_POINT('Ctrl Pts',(0.347078053061478,-0.96052525347768,
0.898302765458188));
#13110=CARTESIAN_POINT('Ctrl Pts',(0.349303707759805,-0.958307704298137,
0.940770468670701));
#13111=CARTESIAN_POINT('Ctrl Pts',(0.351529312469145,-0.956090135383351,
0.983238173449507));
#13112=CARTESIAN_POINT('Ctrl Pts',(0.35375496723721,-0.953872602525604,
1.02570587749755));
#13113=CARTESIAN_POINT('Ctrl Pts',(0.346998431491642,-0.931328747842296,
0.896783495400846));
#13114=CARTESIAN_POINT('Ctrl Pts',(0.349224074223285,-0.929112823219098,
0.939251288581378));
#13115=CARTESIAN_POINT('Ctrl Pts',(0.3514497169821,-0.926896908559584,0.98171908228038));
#13116=CARTESIAN_POINT('Ctrl Pts',(0.35367535976817,-0.924681003894255,
1.02418687649944));
#13117=CARTESIAN_POINT('',(0.466583029361856,-1.07784922788182,0.9));
#13118=CARTESIAN_POINT('Ctrl Pts',(0.347167001354737,-0.931160914046453,
0.9));
#13119=CARTESIAN_POINT('Ctrl Pts',(0.34716700178392,-0.941918922633709,
0.89999999999014));
#13120=CARTESIAN_POINT('Ctrl Pts',(0.348348457226296,-0.952625037179515,
0.899998920330619));
#13121=CARTESIAN_POINT('Ctrl Pts',(0.350635026118381,-0.963095666025449,
0.899998881610567));
#13122=CARTESIAN_POINT('Ctrl Pts',(0.352503737518513,-0.971652846855939,
0.899998849966385));
#13123=CARTESIAN_POINT('Ctrl Pts',(0.355111758040853,-0.980053468583104,
0.899999488623984));
#13124=CARTESIAN_POINT('Ctrl Pts',(0.358442500181925,-0.988191468018609,
0.900000335306729));
#13125=CARTESIAN_POINT('Ctrl Pts',(0.362154764014137,-0.997261639077022,
0.900001278973215));
#13126=CARTESIAN_POINT('Ctrl Pts',(0.366728534310471,-1.00591832418384,
0.900002536038328));
#13127=CARTESIAN_POINT('Ctrl Pts',(0.372121756320194,-1.01402249383533,
0.900001139180886));
#13128=CARTESIAN_POINT('Ctrl Pts',(0.377460617198322,-1.02204497728291,
0.899999756403108));
#13129=CARTESIAN_POINT('Ctrl Pts',(0.383603173789776,-1.02952688289601,
0.899995781932517));
#13130=CARTESIAN_POINT('Ctrl Pts',(0.390441954151244,-1.03639066990207,
0.899992822880961));
#13131=CARTESIAN_POINT('Ctrl Pts',(0.398043576670582,-1.0440200884702,0.899989533757499));
#13132=CARTESIAN_POINT('Ctrl Pts',(0.406433719974705,-1.0508151602132,0.89998759991803));
#13133=CARTESIAN_POINT('Ctrl Pts',(0.415453314813275,-1.05667842789903,
0.899988256654353));
#13134=CARTESIAN_POINT('Ctrl Pts',(0.418717986328798,-1.05880065659603,
0.899988494362188));
#13135=CARTESIAN_POINT('Ctrl Pts',(0.422065457324696,-1.0608004431648,0.89998903479261));
#13136=CARTESIAN_POINT('Ctrl Pts',(0.425489105966494,-1.06267176343868,
0.899989815051126));
#13137=CARTESIAN_POINT('Ctrl Pts',(0.434878177994434,-1.06780370385578,
0.899991954845297));
#13138=CARTESIAN_POINT('Ctrl Pts',(0.444763746614507,-1.07193185662919,
0.899996125260102));
#13139=CARTESIAN_POINT('Ctrl Pts',(0.455000483828058,-1.07494865668414,
0.899998508040168));
#13140=CARTESIAN_POINT('Ctrl Pts',(0.458814676066972,-1.07607271165555,
0.899999395860286));
#13141=CARTESIAN_POINT('Ctrl Pts',(0.462677844602733,-1.07704202188211,
0.899999999981245));
#13142=CARTESIAN_POINT('Ctrl Pts',(0.466583029361856,-1.07784922788182,
0.9));
#13143=CARTESIAN_POINT('Ctrl Pts',(0.466583029361855,-1.07784922788182,
0.9));
#13144=CARTESIAN_POINT('Ctrl Pts',(0.468754418912838,-1.07567408410356,
0.941642632722455));
#13145=CARTESIAN_POINT('Ctrl Pts',(0.470925796725269,-1.07349894615889,
0.983285266331777));
#13146=CARTESIAN_POINT('Ctrl Pts',(0.473097162761967,-1.07132381406029,
1.02492790083044));
#13147=CARTESIAN_POINT('Ctrl Pts',(11.6530064742455,-1.11818194708322,0.896689888359234));
#13148=CARTESIAN_POINT('Ctrl Pts',(11.6507791962577,-1.11596021050721,0.93918888408639));
#13149=CARTESIAN_POINT('Ctrl Pts',(11.6485519182532,-1.11373848005435,0.98168788013277));
#13150=CARTESIAN_POINT('Ctrl Pts',(11.6463246402318,-1.11151675574497,1.02418687649944));
#13151=CARTESIAN_POINT('Ctrl Pts',(11.6528923732761,-1.15994294490385,0.898867064552409));
#13152=CARTESIAN_POINT('Ctrl Pts',(11.6506650597175,-1.15772003758575,0.94136599317676));
#13153=CARTESIAN_POINT('Ctrl Pts',(11.6484378630123,-1.15549719156343,0.98386493116262));
#13154=CARTESIAN_POINT('Ctrl Pts',(11.646210549347,-1.15327429380451,1.02636386026838));
#13155=CARTESIAN_POINT('Ctrl Pts',(11.6202781937939,-1.23241532269502,0.900946494593638));
#13156=CARTESIAN_POINT('Ctrl Pts',(11.6180528194216,-1.23019050716461,0.943445418126786));
#13157=CARTESIAN_POINT('Ctrl Pts',(11.61582741935,-1.22796567893144,0.985944339620759));
#13158=CARTESIAN_POINT('Ctrl Pts',(11.6136020491686,-1.22574086850162,1.02844326360542));
#13159=CARTESIAN_POINT('Ctrl Pts',(11.5499778903249,-1.26376827666489,0.89890126240954));
#13160=CARTESIAN_POINT('Ctrl Pts',(11.5477556460229,-1.26154471817669,0.941400412665532));
#13161=CARTESIAN_POINT('Ctrl Pts',(11.5455333818837,-1.25932119531825,0.983899563748029));
#13162=CARTESIAN_POINT('Ctrl Pts',(11.5433111490058,-1.25709764437074,1.02639871495137));
#13163=CARTESIAN_POINT('Ctrl Pts',(11.5188280133912,-1.26711852942379,0.897443909004722));
#13164=CARTESIAN_POINT('Ctrl Pts',(11.5166067518272,-1.2648961465915,0.93994317191011));
#13165=CARTESIAN_POINT('Ctrl Pts',(11.5143854971699,-1.26267376877071,0.982442435415857));
#13166=CARTESIAN_POINT('Ctrl Pts',(11.512164249443,-1.26045139597664,1.02494169952389));
#13167=CARTESIAN_POINT('',(11.518694417043,-1.26698486563531,0.9));
#13168=CARTESIAN_POINT('Ctrl Pts',(11.5121826600865,-1.26046981594517,1.02458944759559));
#13169=CARTESIAN_POINT('Ctrl Pts',(11.5143532391283,-1.26264149437998,0.983059631155874));
#13170=CARTESIAN_POINT('Ctrl Pts',(11.5165238247878,-1.26481317761477,0.941529815291278));
#13171=CARTESIAN_POINT('Ctrl Pts',(11.518694417043,-1.26698486563531,0.900000000000001));
#13172=CARTESIAN_POINT('Ctrl Pts',(11.518694417043,-1.26698486563531,0.9));
#13173=CARTESIAN_POINT('Ctrl Pts',(11.5293907449245,-1.26586333143554,0.89999999999772));
#13174=CARTESIAN_POINT('Ctrl Pts',(11.5399108669542,-1.26356499290392,0.899998338215302));
#13175=CARTESIAN_POINT('Ctrl Pts',(11.5500820708623,-1.26019169516113,0.899997799246518));
#13176=CARTESIAN_POINT('Ctrl Pts',(11.5583854467913,-1.257437865867,0.899997359253331));
#13177=CARTESIAN_POINT('Ctrl Pts',(11.5664568733073,-1.25396634382171,0.899997630752438));
#13178=CARTESIAN_POINT('Ctrl Pts',(11.5741940388996,-1.24980829733595,0.899998424072895));
#13179=CARTESIAN_POINT('Ctrl Pts',(11.5836658766397,-1.2447180170313,0.899999395255759));
#13180=CARTESIAN_POINT('Ctrl Pts',(11.5925370694996,-1.23865400393036,0.900001263097414));
#13181=CARTESIAN_POINT('Ctrl Pts',(11.6006317325417,-1.23169548876955,0.900000312360774));
#13182=CARTESIAN_POINT('Ctrl Pts',(11.6015335603822,-1.23092023936527,0.900000206439036));
#13183=CARTESIAN_POINT('Ctrl Pts',(11.602425722662,-1.23013384139825,0.900000061718141));
#13184=CARTESIAN_POINT('Ctrl Pts',(11.6033079529217,-1.22933637123764,0.899999870107331));
#13185=CARTESIAN_POINT('Ctrl Pts',(11.6088666967428,-1.22431168263841,0.899998662808674));
#13186=CARTESIAN_POINT('Ctrl Pts',(11.6140319692072,-1.21884801843051,0.89999566823453));
#13187=CARTESIAN_POINT('Ctrl Pts',(11.6187763833168,-1.21300082485405,0.899992820294732));
#13188=CARTESIAN_POINT('Ctrl Pts',(11.6255647330688,-1.20463460846846,0.899988745437233));
#13189=CARTESIAN_POINT('Ctrl Pts',(11.6314252437734,-1.1955686993246,0.899985180772245));
#13190=CARTESIAN_POINT('Ctrl Pts',(11.6362963259193,-1.18598144606113,0.899984461491908));
#13191=CARTESIAN_POINT('Ctrl Pts',(11.6391835002004,-1.18029891593343,0.899984035162064));
#13192=CARTESIAN_POINT('Ctrl Pts',(11.6417223485433,-1.1744324689719,0.89998453059116));
#13193=CARTESIAN_POINT('Ctrl Pts',(11.6438924319112,-1.16841525789854,0.899985826675912));
#13194=CARTESIAN_POINT('Ctrl Pts',(11.6475288754212,-1.15833212078062,0.899987998545922));
#13195=CARTESIAN_POINT('Ctrl Pts',(11.650098554646,-1.1479202064002,0.899992549671115));
#13196=CARTESIAN_POINT('Ctrl Pts',(11.6515257507029,-1.13734249630077,0.899996116295739));
#13197=CARTESIAN_POINT('Ctrl Pts',(11.6523885972688,-1.13094748084967,0.899998272586596));
#13198=CARTESIAN_POINT('Ctrl Pts',(11.6528329982118,-1.12449140232308,0.899999999966183));
#13199=CARTESIAN_POINT('Ctrl Pts',(11.6528329986453,-1.11800890309831,0.9));
#13200=CARTESIAN_POINT('Origin',(6.08275255467124,0.,0.9));
#13201=CARTESIAN_POINT('Ctrl Pts',(11.518694417043,-1.26698486563531,0.9));
#13202=CARTESIAN_POINT('Ctrl Pts',(7.83465728781595,-1.65326443611903,0.9));
#13203=CARTESIAN_POINT('Ctrl Pts',(4.1506201585889,-1.83934349355009,0.9));
#13204=CARTESIAN_POINT('Ctrl Pts',(0.466583029361856,-1.07784922788182,
0.9));
#13205=CARTESIAN_POINT('Ctrl Pts',(11.518694417043,-1.26698486563531,0.9));
#13206=CARTESIAN_POINT('Ctrl Pts',(11.516563806181,-1.26480246768431,0.941642633610146));
#13207=CARTESIAN_POINT('Ctrl Pts',(11.514433195319,-1.2626200697333,0.983285267220291));
#13208=CARTESIAN_POINT('Ctrl Pts',(11.512302584457,-1.2604376717823,1.02492790083044));
#13209=CARTESIAN_POINT('Ctrl Pts',(7.83465728781595,-1.65326443611903,0.9));
#13210=CARTESIAN_POINT('Ctrl Pts',(7.83394897884827,-1.65108203816803,0.941642633610146));
#13211=CARTESIAN_POINT('Ctrl Pts',(7.83324066988059,-1.64889964021702,0.983285267220291));
#13212=CARTESIAN_POINT('Ctrl Pts',(7.83253236091292,-1.64671724226602,1.02492790083044));
#13213=CARTESIAN_POINT('Ctrl Pts',(4.1506201585889,-1.8393434935501,0.9));
#13214=CARTESIAN_POINT('Ctrl Pts',(4.15133415151555,-1.83716109559909,0.941642633610146));
#13215=CARTESIAN_POINT('Ctrl Pts',(4.15204814444219,-1.83497869764808,0.983285267220291));
#13216=CARTESIAN_POINT('Ctrl Pts',(4.15276213736883,-1.83279629969708,1.02492790083044));
#13217=CARTESIAN_POINT('Ctrl Pts',(0.466583029361856,-1.07784922788182,
0.9));
#13218=CARTESIAN_POINT('Ctrl Pts',(0.468719324182819,-1.07566682993082,
0.941642633610146));
#13219=CARTESIAN_POINT('Ctrl Pts',(0.470855619003783,-1.07348443197981,
0.983285267220291));
#13220=CARTESIAN_POINT('Ctrl Pts',(0.472991913824746,-1.07130203402881,
1.02492790083044));
#18337=UNCERTAINTY_MEASURE_WITH_UNIT(LENGTH_MEASURE(0.001),#18354,
'DISTANCE_ACCURACY_VALUE',
'Maximum model space distance between geometric entities at asserted c
onnectivities');
#18341=UNCERTAINTY_MEASURE_WITH_UNIT(LENGTH_MEASURE(0.001),#18354,
'DISTANCE_ACCURACY_VALUE',
'Maximum model space distance between geometric entities at asserted c
onnectivities');
#18349=(
GEOMETRIC_REPRESENTATION_CONTEXT(3)
GLOBAL_UNCERTAINTY_ASSIGNED_CONTEXT((#18337))
GLOBAL_UNIT_ASSIGNED_CONTEXT((#18354,#18356,#18357))
REPRESENTATION_CONTEXT('','3D')
);
#18353=(
GEOMETRIC_REPRESENTATION_CONTEXT(3)
GLOBAL_UNCERTAINTY_ASSIGNED_CONTEXT((#18341))
GLOBAL_UNIT_ASSIGNED_CONTEXT((#18354,#18356,#18357))
REPRESENTATION_CONTEXT('','3D')
);
#18354=(
LENGTH_UNIT()
NAMED_UNIT(*)
SI_UNIT(.CENTI.,.METRE.)
);
#18356=(
NAMED_UNIT(*)
PLANE_ANGLE_UNIT()
SI_UNIT($,.RADIAN.)
);
#18357=(
NAMED_UNIT(*)
SI_UNIT($,.STERADIAN.)
SOLID_ANGLE_UNIT()
);
#18365=SHAPE_DEFINITION_REPRESENTATION(#18376,#18403);
#18376=PRODUCT_DEFINITION_SHAPE('',$,#18415);
#18403=SHAPE_REPRESENTATION('',(#6896),#18349);
#18407=PRODUCT_DEFINITION_CONTEXT('part definition',#18442,'design');
#18415=PRODUCT_DEFINITION('2026-11-10-01-32-12-364','Soft grip layer',#18426,
#18407);
#18426=PRODUCT_DEFINITION_FORMATION('',$,#18451);
#18442=APPLICATION_CONTEXT(
'Core Data for Automotive Mechanical Design Process');
#18443=PRODUCT_CONTEXT('part definition',#18442,'mechanical');
#18451=PRODUCT('2026-11-10-01-32-12-364','Soft grip layer',$,(#18443));
#18460=PRESENTATION_STYLE_ASSIGNMENT((#18468));
#18468=SURFACE_STYLE_USAGE(.BOTH.,#18476);
#18476=SURFACE_SIDE_STYLE('',(#18484));
#18484=SURFACE_STYLE_FILL_AREA(#18492);
#18492=FILL_AREA_STYLE('Sky blue soft grip',(#18500));
#18500=FILL_AREA_STYLE_COLOUR('Sky blue soft grip',#18508);
#18508=COLOUR_RGB('Sky blue soft grip',0.662745098039216,0.831372549019608,
0.949019607843137);
ENDSEC;
END-ISO-10303-21;
